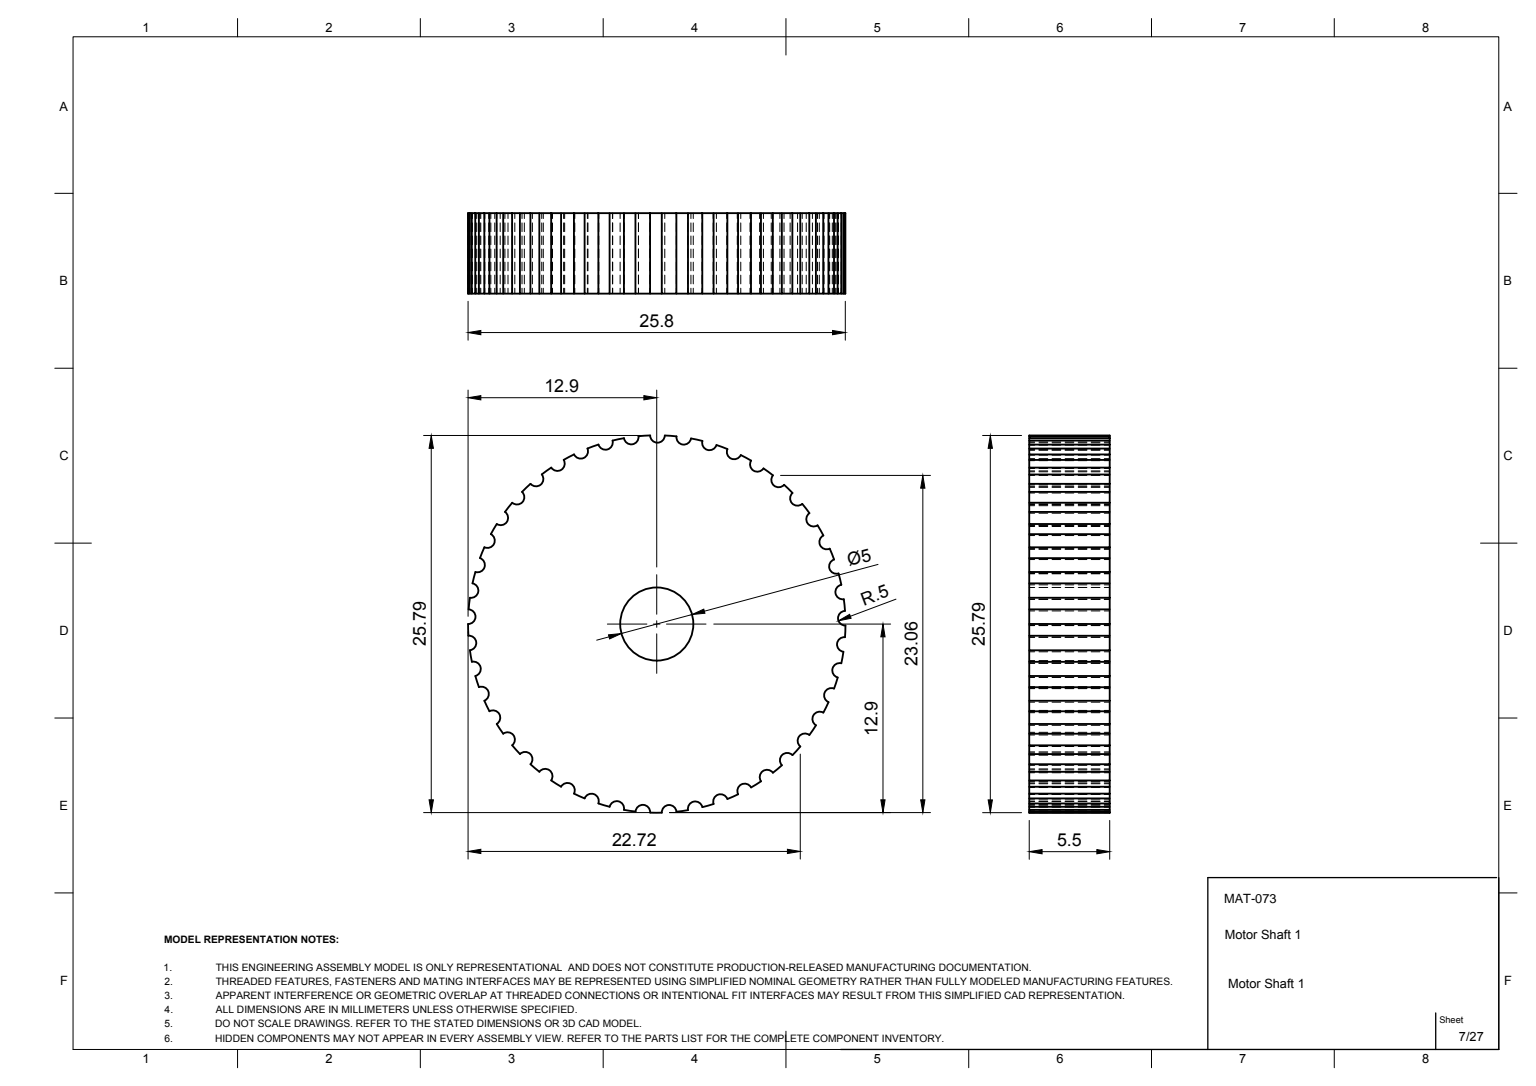
ISO-10303-21;
HEADER;
/* Generated by software containing ST-Developer
 * from STEP Tools, Inc. (www.steptools.com) 
 */

FILE_DESCRIPTION(
/* description */ ('CAx-IF Rec.Pracs.---Representation and Presentation of Product Manufa
cturing Information (PMI)---4.0---2014-10-13'),
/* implementation_level */ '2;1');

FILE_NAME(
/* name */ 'Motor Shaft 1.step',
/* time_stamp */ '2026-10-24T18:52:33-07:00',
/* author */ (''),
/* organization */ (''),
/* preprocessor_version */ 'ST-DEVELOPER v20.2',
/* originating_system */ 'Autodesk Translation Framework v15.17.0.0',
/* authorisation */ '');

FILE_SCHEMA (('AP242_MANAGED_MODEL_BASED_3D_ENGINEERING_MIM_LF { 1 0 10303 442 2 1 4 }'));
ENDSEC;

DATA;
#10=MECHANICAL_DESIGN_GEOMETRIC_PRESENTATION_REPRESENTATION('',(#418),#34876);
#352=SHAPE_REPRESENTATION_RELATIONSHIP('SRR','None',#34989,#385);
#385=ADVANCED_BREP_SHAPE_REPRESENTATION('',(#451),#34847);
#418=STYLED_ITEM('',(#35163),#451);
#451=MANIFOLD_SOLID_BREP('Motor Shaft 1',#19558);
#501=FACE_BOUND('',#6091,.T.);
#502=FACE_BOUND('',#6138,.T.);
#717=PLANE('',#20448);
#718=PLANE('',#20586);
#1387=LINE('',#29757,#2986);
#1388=LINE('',#29761,#2987);
#1389=LINE('',#29766,#2988);
#1390=LINE('',#29770,#2989);
#1391=LINE('',#29775,#2990);
#1392=LINE('',#29779,#2991);
#1393=LINE('',#29784,#2992);
#1394=LINE('',#29788,#2993);
#1395=LINE('',#29793,#2994);
#1396=LINE('',#29797,#2995);
#1397=LINE('',#29802,#2996);
#1398=LINE('',#29806,#2997);
#1399=LINE('',#29811,#2998);
#1400=LINE('',#29815,#2999);
#1401=LINE('',#29820,#3000);
#1402=LINE('',#29824,#3001);
#1403=LINE('',#29829,#3002);
#1404=LINE('',#29833,#3003);
#1405=LINE('',#29838,#3004);
#1406=LINE('',#29842,#3005);
#1407=LINE('',#29847,#3006);
#1408=LINE('',#29851,#3007);
#1409=LINE('',#29856,#3008);
#1410=LINE('',#29860,#3009);
#1411=LINE('',#29865,#3010);
#1412=LINE('',#29869,#3011);
#1413=LINE('',#29874,#3012);
#1414=LINE('',#29878,#3013);
#1415=LINE('',#29883,#3014);
#1416=LINE('',#29887,#3015);
#1417=LINE('',#29892,#3016);
#1418=LINE('',#29896,#3017);
#1419=LINE('',#29901,#3018);
#1420=LINE('',#29905,#3019);
#1421=LINE('',#29910,#3020);
#1422=LINE('',#29914,#3021);
#1423=LINE('',#29919,#3022);
#1424=LINE('',#29923,#3023);
#1425=LINE('',#29928,#3024);
#1426=LINE('',#29932,#3025);
#1427=LINE('',#29937,#3026);
#1428=LINE('',#29941,#3027);
#1429=LINE('',#29946,#3028);
#1430=LINE('',#29950,#3029);
#1431=LINE('',#29955,#3030);
#1432=LINE('',#29959,#3031);
#1433=LINE('',#29964,#3032);
#1434=LINE('',#29968,#3033);
#1435=LINE('',#29973,#3034);
#1436=LINE('',#29977,#3035);
#1437=LINE('',#29982,#3036);
#1438=LINE('',#29986,#3037);
#1439=LINE('',#29991,#3038);
#1440=LINE('',#29995,#3039);
#1441=LINE('',#30000,#3040);
#1442=LINE('',#30004,#3041);
#1443=LINE('',#30009,#3042);
#1444=LINE('',#30013,#3043);
#1445=LINE('',#30018,#3044);
#1446=LINE('',#30022,#3045);
#1447=LINE('',#30027,#3046);
#1448=LINE('',#30031,#3047);
#1449=LINE('',#30036,#3048);
#1450=LINE('',#30040,#3049);
#1451=LINE('',#30045,#3050);
#1452=LINE('',#30049,#3051);
#1453=LINE('',#30054,#3052);
#1454=LINE('',#30058,#3053);
#1455=LINE('',#30063,#3054);
#1456=LINE('',#30067,#3055);
#1457=LINE('',#30072,#3056);
#1458=LINE('',#30076,#3057);
#1459=LINE('',#30081,#3058);
#1460=LINE('',#30085,#3059);
#1461=LINE('',#30090,#3060);
#1462=LINE('',#30094,#3061);
#1463=LINE('',#30099,#3062);
#1464=LINE('',#30103,#3063);
#1465=LINE('',#30108,#3064);
#1466=LINE('',#30112,#3065);
#1467=LINE('',#30117,#3066);
#1468=LINE('',#30121,#3067);
#1469=LINE('',#30126,#3068);
#1470=LINE('',#30130,#3069);
#1471=LINE('',#30135,#3070);
#1472=LINE('',#30139,#3071);
#1473=LINE('',#30144,#3072);
#1474=LINE('',#30148,#3073);
#1475=LINE('',#30204,#3074);
#1476=LINE('',#30207,#3075);
#1477=LINE('',#30301,#3076);
#2986=VECTOR('',#23294,1.);
#2987=VECTOR('',#23297,1.);
#2988=VECTOR('',#23302,1.);
#2989=VECTOR('',#23305,1.);
#2990=VECTOR('',#23310,1.);
#2991=VECTOR('',#23313,1.);
#2992=VECTOR('',#23318,1.);
#2993=VECTOR('',#23321,1.);
#2994=VECTOR('',#23326,1.);
#2995=VECTOR('',#23329,1.);
#2996=VECTOR('',#23334,1.);
#2997=VECTOR('',#23337,1.);
#2998=VECTOR('',#23342,1.);
#2999=VECTOR('',#23345,1.);
#3000=VECTOR('',#23350,1.);
#3001=VECTOR('',#23353,1.);
#3002=VECTOR('',#23358,1.);
#3003=VECTOR('',#23361,1.);
#3004=VECTOR('',#23366,1.);
#3005=VECTOR('',#23369,1.);
#3006=VECTOR('',#23374,1.);
#3007=VECTOR('',#23377,1.);
#3008=VECTOR('',#23382,1.);
#3009=VECTOR('',#23385,1.);
#3010=VECTOR('',#23390,1.);
#3011=VECTOR('',#23393,1.);
#3012=VECTOR('',#23398,1.);
#3013=VECTOR('',#23401,1.);
#3014=VECTOR('',#23406,1.);
#3015=VECTOR('',#23409,1.);
#3016=VECTOR('',#23414,1.);
#3017=VECTOR('',#23417,1.);
#3018=VECTOR('',#23422,1.);
#3019=VECTOR('',#23425,1.);
#3020=VECTOR('',#23430,1.);
#3021=VECTOR('',#23433,1.);
#3022=VECTOR('',#23438,1.);
#3023=VECTOR('',#23441,1.);
#3024=VECTOR('',#23446,1.);
#3025=VECTOR('',#23449,1.);
#3026=VECTOR('',#23454,1.);
#3027=VECTOR('',#23457,1.);
#3028=VECTOR('',#23462,1.);
#3029=VECTOR('',#23465,1.);
#3030=VECTOR('',#23470,1.);
#3031=VECTOR('',#23473,1.);
#3032=VECTOR('',#23478,1.);
#3033=VECTOR('',#23481,1.);
#3034=VECTOR('',#23486,1.);
#3035=VECTOR('',#23489,1.);
#3036=VECTOR('',#23494,1.);
#3037=VECTOR('',#23497,1.);
#3038=VECTOR('',#23502,1.);
#3039=VECTOR('',#23505,1.);
#3040=VECTOR('',#23510,1.);
#3041=VECTOR('',#23513,1.);
#3042=VECTOR('',#23518,1.);
#3043=VECTOR('',#23521,1.);
#3044=VECTOR('',#23526,1.);
#3045=VECTOR('',#23529,1.);
#3046=VECTOR('',#23534,1.);
#3047=VECTOR('',#23537,1.);
#3048=VECTOR('',#23542,1.);
#3049=VECTOR('',#23545,1.);
#3050=VECTOR('',#23550,1.);
#3051=VECTOR('',#23553,1.);
#3052=VECTOR('',#23558,1.);
#3053=VECTOR('',#23561,1.);
#3054=VECTOR('',#23566,1.);
#3055=VECTOR('',#23569,1.);
#3056=VECTOR('',#23574,1.);
#3057=VECTOR('',#23577,1.);
#3058=VECTOR('',#23582,1.);
#3059=VECTOR('',#23585,1.);
#3060=VECTOR('',#23590,1.);
#3061=VECTOR('',#23593,1.);
#3062=VECTOR('',#23598,1.);
#3063=VECTOR('',#23601,1.);
#3064=VECTOR('',#23606,1.);
#3065=VECTOR('',#23609,1.);
#3066=VECTOR('',#23614,1.);
#3067=VECTOR('',#23617,1.);
#3068=VECTOR('',#23622,1.);
#3069=VECTOR('',#23625,1.);
#3070=VECTOR('',#23630,1.);
#3071=VECTOR('',#23633,1.);
#3072=VECTOR('',#23638,1.);
#3073=VECTOR('',#23641,1.);
#3074=VECTOR('',#23744,1.);
#3075=VECTOR('',#23747,1.);
#3076=VECTOR('',#23932,0.0025);
#4339=CYLINDRICAL_SURFACE('',#20316,0.0005);
#4340=CYLINDRICAL_SURFACE('',#20319,0.0005);
#4341=CYLINDRICAL_SURFACE('',#20322,0.0005);
#4342=CYLINDRICAL_SURFACE('',#20325,0.0005);
#4343=CYLINDRICAL_SURFACE('',#20328,0.0005);
#4344=CYLINDRICAL_SURFACE('',#20331,0.0005);
#4345=CYLINDRICAL_SURFACE('',#20334,0.0005);
#4346=CYLINDRICAL_SURFACE('',#20337,0.0005);
#4347=CYLINDRICAL_SURFACE('',#20340,0.0005);
#4348=CYLINDRICAL_SURFACE('',#20343,0.0005);
#4349=CYLINDRICAL_SURFACE('',#20346,0.0005);
#4350=CYLINDRICAL_SURFACE('',#20349,0.0005);
#4351=CYLINDRICAL_SURFACE('',#20352,0.0005);
#4352=CYLINDRICAL_SURFACE('',#20355,0.0005);
#4353=CYLINDRICAL_SURFACE('',#20358,0.0005);
#4354=CYLINDRICAL_SURFACE('',#20361,0.0005);
#4355=CYLINDRICAL_SURFACE('',#20364,0.0005);
#4356=CYLINDRICAL_SURFACE('',#20367,0.0005);
#4357=CYLINDRICAL_SURFACE('',#20370,0.0005);
#4358=CYLINDRICAL_SURFACE('',#20373,0.0005);
#4359=CYLINDRICAL_SURFACE('',#20376,0.0005);
#4360=CYLINDRICAL_SURFACE('',#20379,0.0005);
#4361=CYLINDRICAL_SURFACE('',#20382,0.0005);
#4362=CYLINDRICAL_SURFACE('',#20385,0.0005);
#4363=CYLINDRICAL_SURFACE('',#20388,0.0005);
#4364=CYLINDRICAL_SURFACE('',#20391,0.0005);
#4365=CYLINDRICAL_SURFACE('',#20394,0.0005);
#4366=CYLINDRICAL_SURFACE('',#20397,0.0005);
#4367=CYLINDRICAL_SURFACE('',#20400,0.0005);
#4368=CYLINDRICAL_SURFACE('',#20403,0.0005);
#4369=CYLINDRICAL_SURFACE('',#20406,0.0005);
#4370=CYLINDRICAL_SURFACE('',#20409,0.0005);
#4371=CYLINDRICAL_SURFACE('',#20412,0.0005);
#4372=CYLINDRICAL_SURFACE('',#20415,0.0005);
#4373=CYLINDRICAL_SURFACE('',#20418,0.0005);
#4374=CYLINDRICAL_SURFACE('',#20421,0.0005);
#4375=CYLINDRICAL_SURFACE('',#20424,0.0005);
#4376=CYLINDRICAL_SURFACE('',#20427,0.0005);
#4377=CYLINDRICAL_SURFACE('',#20430,0.0005);
#4378=CYLINDRICAL_SURFACE('',#20433,0.0005);
#4379=CYLINDRICAL_SURFACE('',#20436,0.0005);
#4380=CYLINDRICAL_SURFACE('',#20439,0.0005);
#4381=CYLINDRICAL_SURFACE('',#20442,0.0005);
#4382=CYLINDRICAL_SURFACE('',#20445,0.0005);
#4383=CYLINDRICAL_SURFACE('',#20496,0.0129);
#4384=CYLINDRICAL_SURFACE('',#20498,0.0129);
#4385=CYLINDRICAL_SURFACE('',#20500,0.0129);
#4386=CYLINDRICAL_SURFACE('',#20502,0.0129);
#4387=CYLINDRICAL_SURFACE('',#20504,0.0129);
#4388=CYLINDRICAL_SURFACE('',#20506,0.0129);
#4389=CYLINDRICAL_SURFACE('',#20508,0.0129);
#4390=CYLINDRICAL_SURFACE('',#20510,0.0129);
#4391=CYLINDRICAL_SURFACE('',#20512,0.0129);
#4392=CYLINDRICAL_SURFACE('',#20514,0.0129);
#4393=CYLINDRICAL_SURFACE('',#20516,0.0129);
#4394=CYLINDRICAL_SURFACE('',#20518,0.0129);
#4395=CYLINDRICAL_SURFACE('',#20520,0.0129);
#4396=CYLINDRICAL_SURFACE('',#20522,0.0129);
#4397=CYLINDRICAL_SURFACE('',#20524,0.0129);
#4398=CYLINDRICAL_SURFACE('',#20526,0.0129);
#4399=CYLINDRICAL_SURFACE('',#20528,0.0129);
#4400=CYLINDRICAL_SURFACE('',#20530,0.0129);
#4401=CYLINDRICAL_SURFACE('',#20532,0.0129);
#4402=CYLINDRICAL_SURFACE('',#20534,0.0129);
#4403=CYLINDRICAL_SURFACE('',#20536,0.0129);
#4404=CYLINDRICAL_SURFACE('',#20538,0.0129);
#4405=CYLINDRICAL_SURFACE('',#20540,0.0129);
#4406=CYLINDRICAL_SURFACE('',#20542,0.0129);
#4407=CYLINDRICAL_SURFACE('',#20544,0.0129);
#4408=CYLINDRICAL_SURFACE('',#20546,0.0129);
#4409=CYLINDRICAL_SURFACE('',#20548,0.0129);
#4410=CYLINDRICAL_SURFACE('',#20550,0.0129);
#4411=CYLINDRICAL_SURFACE('',#20552,0.0129);
#4412=CYLINDRICAL_SURFACE('',#20554,0.0129);
#4413=CYLINDRICAL_SURFACE('',#20556,0.0129);
#4414=CYLINDRICAL_SURFACE('',#20558,0.0129);
#4415=CYLINDRICAL_SURFACE('',#20560,0.0129);
#4416=CYLINDRICAL_SURFACE('',#20562,0.0129);
#4417=CYLINDRICAL_SURFACE('',#20564,0.0129);
#4418=CYLINDRICAL_SURFACE('',#20566,0.0129);
#4419=CYLINDRICAL_SURFACE('',#20568,0.0129);
#4420=CYLINDRICAL_SURFACE('',#20570,0.0129);
#4421=CYLINDRICAL_SURFACE('',#20572,0.0129);
#4422=CYLINDRICAL_SURFACE('',#20574,0.0129);
#4423=CYLINDRICAL_SURFACE('',#20576,0.0129);
#4424=CYLINDRICAL_SURFACE('',#20578,0.0129);
#4425=CYLINDRICAL_SURFACE('',#20580,0.0129);
#4426=CYLINDRICAL_SURFACE('',#20582,0.0129);
#4427=CYLINDRICAL_SURFACE('',#20584,0.0005);
#4428=CYLINDRICAL_SURFACE('',#20589,0.0129);
#4429=CYLINDRICAL_SURFACE('',#20590,0.0025);
#4980=FACE_OUTER_BOUND('',#6046,.T.);
#4981=FACE_OUTER_BOUND('',#6047,.T.);
#4982=FACE_OUTER_BOUND('',#6048,.T.);
#4983=FACE_OUTER_BOUND('',#6049,.T.);
#4984=FACE_OUTER_BOUND('',#6050,.T.);
#4985=FACE_OUTER_BOUND('',#6051,.T.);
#4986=FACE_OUTER_BOUND('',#6052,.T.);
#4987=FACE_OUTER_BOUND('',#6053,.T.);
#4988=FACE_OUTER_BOUND('',#6054,.T.);
#4989=FACE_OUTER_BOUND('',#6055,.T.);
#4990=FACE_OUTER_BOUND('',#6056,.T.);
#4991=FACE_OUTER_BOUND('',#6057,.T.);
#4992=FACE_OUTER_BOUND('',#6058,.T.);
#4993=FACE_OUTER_BOUND('',#6059,.T.);
#4994=FACE_OUTER_BOUND('',#6060,.T.);
#4995=FACE_OUTER_BOUND('',#6061,.T.);
#4996=FACE_OUTER_BOUND('',#6062,.T.);
#4997=FACE_OUTER_BOUND('',#6063,.T.);
#4998=FACE_OUTER_BOUND('',#6064,.T.);
#4999=FACE_OUTER_BOUND('',#6065,.T.);
#5000=FACE_OUTER_BOUND('',#6066,.T.);
#5001=FACE_OUTER_BOUND('',#6067,.T.);
#5002=FACE_OUTER_BOUND('',#6068,.T.);
#5003=FACE_OUTER_BOUND('',#6069,.T.);
#5004=FACE_OUTER_BOUND('',#6070,.T.);
#5005=FACE_OUTER_BOUND('',#6071,.T.);
#5006=FACE_OUTER_BOUND('',#6072,.T.);
#5007=FACE_OUTER_BOUND('',#6073,.T.);
#5008=FACE_OUTER_BOUND('',#6074,.T.);
#5009=FACE_OUTER_BOUND('',#6075,.T.);
#5010=FACE_OUTER_BOUND('',#6076,.T.);
#5011=FACE_OUTER_BOUND('',#6077,.T.);
#5012=FACE_OUTER_BOUND('',#6078,.T.);
#5013=FACE_OUTER_BOUND('',#6079,.T.);
#5014=FACE_OUTER_BOUND('',#6080,.T.);
#5015=FACE_OUTER_BOUND('',#6081,.T.);
#5016=FACE_OUTER_BOUND('',#6082,.T.);
#5017=FACE_OUTER_BOUND('',#6083,.T.);
#5018=FACE_OUTER_BOUND('',#6084,.T.);
#5019=FACE_OUTER_BOUND('',#6085,.T.);
#5020=FACE_OUTER_BOUND('',#6086,.T.);
#5021=FACE_OUTER_BOUND('',#6087,.T.);
#5022=FACE_OUTER_BOUND('',#6088,.T.);
#5023=FACE_OUTER_BOUND('',#6089,.T.);
#5024=FACE_OUTER_BOUND('',#6090,.T.);
#5025=FACE_OUTER_BOUND('',#6092,.T.);
#5026=FACE_OUTER_BOUND('',#6093,.T.);
#5027=FACE_OUTER_BOUND('',#6094,.T.);
#5028=FACE_OUTER_BOUND('',#6095,.T.);
#5029=FACE_OUTER_BOUND('',#6096,.T.);
#5030=FACE_OUTER_BOUND('',#6097,.T.);
#5031=FACE_OUTER_BOUND('',#6098,.T.);
#5032=FACE_OUTER_BOUND('',#6099,.T.);
#5033=FACE_OUTER_BOUND('',#6100,.T.);
#5034=FACE_OUTER_BOUND('',#6101,.T.);
#5035=FACE_OUTER_BOUND('',#6102,.T.);
#5036=FACE_OUTER_BOUND('',#6103,.T.);
#5037=FACE_OUTER_BOUND('',#6104,.T.);
#5038=FACE_OUTER_BOUND('',#6105,.T.);
#5039=FACE_OUTER_BOUND('',#6106,.T.);
#5040=FACE_OUTER_BOUND('',#6107,.T.);
#5041=FACE_OUTER_BOUND('',#6108,.T.);
#5042=FACE_OUTER_BOUND('',#6109,.T.);
#5043=FACE_OUTER_BOUND('',#6110,.T.);
#5044=FACE_OUTER_BOUND('',#6111,.T.);
#5045=FACE_OUTER_BOUND('',#6112,.T.);
#5046=FACE_OUTER_BOUND('',#6113,.T.);
#5047=FACE_OUTER_BOUND('',#6114,.T.);
#5048=FACE_OUTER_BOUND('',#6115,.T.);
#5049=FACE_OUTER_BOUND('',#6116,.T.);
#5050=FACE_OUTER_BOUND('',#6117,.T.);
#5051=FACE_OUTER_BOUND('',#6118,.T.);
#5052=FACE_OUTER_BOUND('',#6119,.T.);
#5053=FACE_OUTER_BOUND('',#6120,.T.);
#5054=FACE_OUTER_BOUND('',#6121,.T.);
#5055=FACE_OUTER_BOUND('',#6122,.T.);
#5056=FACE_OUTER_BOUND('',#6123,.T.);
#5057=FACE_OUTER_BOUND('',#6124,.T.);
#5058=FACE_OUTER_BOUND('',#6125,.T.);
#5059=FACE_OUTER_BOUND('',#6126,.T.);
#5060=FACE_OUTER_BOUND('',#6127,.T.);
#5061=FACE_OUTER_BOUND('',#6128,.T.);
#5062=FACE_OUTER_BOUND('',#6129,.T.);
#5063=FACE_OUTER_BOUND('',#6130,.T.);
#5064=FACE_OUTER_BOUND('',#6131,.T.);
#5065=FACE_OUTER_BOUND('',#6132,.T.);
#5066=FACE_OUTER_BOUND('',#6133,.T.);
#5067=FACE_OUTER_BOUND('',#6134,.T.);
#5068=FACE_OUTER_BOUND('',#6135,.T.);
#5069=FACE_OUTER_BOUND('',#6136,.T.);
#5070=FACE_OUTER_BOUND('',#6137,.T.);
#5071=FACE_OUTER_BOUND('',#6139,.T.);
#5072=FACE_OUTER_BOUND('',#6140,.T.);
#6046=EDGE_LOOP('',(#13790,#13791,#13792,#13793));
#6047=EDGE_LOOP('',(#13794,#13795,#13796,#13797));
#6048=EDGE_LOOP('',(#13798,#13799,#13800,#13801));
#6049=EDGE_LOOP('',(#13802,#13803,#13804,#13805));
#6050=EDGE_LOOP('',(#13806,#13807,#13808,#13809));
#6051=EDGE_LOOP('',(#13810,#13811,#13812,#13813));
#6052=EDGE_LOOP('',(#13814,#13815,#13816,#13817));
#6053=EDGE_LOOP('',(#13818,#13819,#13820,#13821));
#6054=EDGE_LOOP('',(#13822,#13823,#13824,#13825));
#6055=EDGE_LOOP('',(#13826,#13827,#13828,#13829));
#6056=EDGE_LOOP('',(#13830,#13831,#13832,#13833));
#6057=EDGE_LOOP('',(#13834,#13835,#13836,#13837));
#6058=EDGE_LOOP('',(#13838,#13839,#13840,#13841));
#6059=EDGE_LOOP('',(#13842,#13843,#13844,#13845));
#6060=EDGE_LOOP('',(#13846,#13847,#13848,#13849));
#6061=EDGE_LOOP('',(#13850,#13851,#13852,#13853));
#6062=EDGE_LOOP('',(#13854,#13855,#13856,#13857));
#6063=EDGE_LOOP('',(#13858,#13859,#13860,#13861));
#6064=EDGE_LOOP('',(#13862,#13863,#13864,#13865));
#6065=EDGE_LOOP('',(#13866,#13867,#13868,#13869));
#6066=EDGE_LOOP('',(#13870,#13871,#13872,#13873));
#6067=EDGE_LOOP('',(#13874,#13875,#13876,#13877));
#6068=EDGE_LOOP('',(#13878,#13879,#13880,#13881));
#6069=EDGE_LOOP('',(#13882,#13883,#13884,#13885));
#6070=EDGE_LOOP('',(#13886,#13887,#13888,#13889));
#6071=EDGE_LOOP('',(#13890,#13891,#13892,#13893));
#6072=EDGE_LOOP('',(#13894,#13895,#13896,#13897));
#6073=EDGE_LOOP('',(#13898,#13899,#13900,#13901));
#6074=EDGE_LOOP('',(#13902,#13903,#13904,#13905));
#6075=EDGE_LOOP('',(#13906,#13907,#13908,#13909));
#6076=EDGE_LOOP('',(#13910,#13911,#13912,#13913));
#6077=EDGE_LOOP('',(#13914,#13915,#13916,#13917));
#6078=EDGE_LOOP('',(#13918,#13919,#13920,#13921));
#6079=EDGE_LOOP('',(#13922,#13923,#13924,#13925));
#6080=EDGE_LOOP('',(#13926,#13927,#13928,#13929));
#6081=EDGE_LOOP('',(#13930,#13931,#13932,#13933));
#6082=EDGE_LOOP('',(#13934,#13935,#13936,#13937));
#6083=EDGE_LOOP('',(#13938,#13939,#13940,#13941));
#6084=EDGE_LOOP('',(#13942,#13943,#13944,#13945));
#6085=EDGE_LOOP('',(#13946,#13947,#13948,#13949));
#6086=EDGE_LOOP('',(#13950,#13951,#13952,#13953));
#6087=EDGE_LOOP('',(#13954,#13955,#13956,#13957));
#6088=EDGE_LOOP('',(#13958,#13959,#13960,#13961));
#6089=EDGE_LOOP('',(#13962,#13963,#13964,#13965));
#6090=EDGE_LOOP('',(#13966,#13967,#13968,#13969,#13970,#13971,#13972,#13973,
#13974,#13975,#13976,#13977,#13978,#13979,#13980,#13981,#13982,#13983,#13984,
#13985,#13986,#13987,#13988,#13989,#13990,#13991,#13992,#13993,#13994,#13995,
#13996,#13997,#13998,#13999,#14000,#14001,#14002,#14003,#14004,#14005,#14006,
#14007,#14008,#14009,#14010,#14011,#14012,#14013,#14014,#14015,#14016,#14017,
#14018,#14019,#14020,#14021,#14022,#14023,#14024,#14025,#14026,#14027,#14028,
#14029,#14030,#14031,#14032,#14033,#14034,#14035,#14036,#14037,#14038,#14039,
#14040,#14041,#14042,#14043,#14044,#14045,#14046,#14047,#14048,#14049,#14050,
#14051,#14052,#14053,#14054,#14055));
#6091=EDGE_LOOP('',(#14056));
#6092=EDGE_LOOP('',(#14057,#14058,#14059,#14060));
#6093=EDGE_LOOP('',(#14061,#14062,#14063,#14064));
#6094=EDGE_LOOP('',(#14065,#14066,#14067,#14068));
#6095=EDGE_LOOP('',(#14069,#14070,#14071,#14072));
#6096=EDGE_LOOP('',(#14073,#14074,#14075,#14076));
#6097=EDGE_LOOP('',(#14077,#14078,#14079,#14080));
#6098=EDGE_LOOP('',(#14081,#14082,#14083,#14084));
#6099=EDGE_LOOP('',(#14085,#14086,#14087,#14088));
#6100=EDGE_LOOP('',(#14089,#14090,#14091,#14092));
#6101=EDGE_LOOP('',(#14093,#14094,#14095,#14096));
#6102=EDGE_LOOP('',(#14097,#14098,#14099,#14100));
#6103=EDGE_LOOP('',(#14101,#14102,#14103,#14104));
#6104=EDGE_LOOP('',(#14105,#14106,#14107,#14108));
#6105=EDGE_LOOP('',(#14109,#14110,#14111,#14112));
#6106=EDGE_LOOP('',(#14113,#14114,#14115,#14116));
#6107=EDGE_LOOP('',(#14117,#14118,#14119,#14120));
#6108=EDGE_LOOP('',(#14121,#14122,#14123,#14124));
#6109=EDGE_LOOP('',(#14125,#14126,#14127,#14128));
#6110=EDGE_LOOP('',(#14129,#14130,#14131,#14132));
#6111=EDGE_LOOP('',(#14133,#14134,#14135,#14136));
#6112=EDGE_LOOP('',(#14137,#14138,#14139,#14140));
#6113=EDGE_LOOP('',(#14141,#14142,#14143,#14144));
#6114=EDGE_LOOP('',(#14145,#14146,#14147,#14148));
#6115=EDGE_LOOP('',(#14149,#14150,#14151,#14152));
#6116=EDGE_LOOP('',(#14153,#14154,#14155,#14156));
#6117=EDGE_LOOP('',(#14157,#14158,#14159,#14160));
#6118=EDGE_LOOP('',(#14161,#14162,#14163,#14164));
#6119=EDGE_LOOP('',(#14165,#14166,#14167,#14168));
#6120=EDGE_LOOP('',(#14169,#14170,#14171,#14172));
#6121=EDGE_LOOP('',(#14173,#14174,#14175,#14176));
#6122=EDGE_LOOP('',(#14177,#14178,#14179,#14180));
#6123=EDGE_LOOP('',(#14181,#14182,#14183,#14184));
#6124=EDGE_LOOP('',(#14185,#14186,#14187,#14188));
#6125=EDGE_LOOP('',(#14189,#14190,#14191,#14192));
#6126=EDGE_LOOP('',(#14193,#14194,#14195,#14196));
#6127=EDGE_LOOP('',(#14197,#14198,#14199,#14200));
#6128=EDGE_LOOP('',(#14201,#14202,#14203,#14204));
#6129=EDGE_LOOP('',(#14205,#14206,#14207,#14208));
#6130=EDGE_LOOP('',(#14209,#14210,#14211,#14212));
#6131=EDGE_LOOP('',(#14213,#14214,#14215,#14216));
#6132=EDGE_LOOP('',(#14217,#14218,#14219,#14220));
#6133=EDGE_LOOP('',(#14221,#14222,#14223,#14224));
#6134=EDGE_LOOP('',(#14225,#14226,#14227,#14228));
#6135=EDGE_LOOP('',(#14229,#14230,#14231,#14232));
#6136=EDGE_LOOP('',(#14233,#14234,#14235,#14236));
#6137=EDGE_LOOP('',(#14237,#14238,#14239,#14240,#14241,#14242,#14243,#14244,
#14245,#14246,#14247,#14248,#14249,#14250,#14251,#14252,#14253,#14254,#14255,
#14256,#14257,#14258,#14259,#14260,#14261,#14262,#14263,#14264,#14265,#14266,
#14267,#14268,#14269,#14270,#14271,#14272,#14273,#14274,#14275,#14276,#14277,
#14278,#14279,#14280,#14281,#14282,#14283,#14284,#14285,#14286,#14287,#14288,
#14289,#14290,#14291,#14292,#14293,#14294,#14295,#14296,#14297,#14298,#14299,
#14300,#14301,#14302,#14303,#14304,#14305,#14306,#14307,#14308,#14309,#14310,
#14311,#14312,#14313,#14314,#14315,#14316,#14317,#14318,#14319,#14320,#14321,
#14322,#14323,#14324,#14325,#14326));
#6138=EDGE_LOOP('',(#14327));
#6139=EDGE_LOOP('',(#14328,#14329,#14330,#14331));
#6140=EDGE_LOOP('',(#14332,#14333,#14334,#14335));
#7101=CIRCLE('',#20317,0.000500000000011295);
#7102=CIRCLE('',#20318,0.000500000000011295);
#7103=CIRCLE('',#20320,0.000500000000012369);
#7104=CIRCLE('',#20321,0.000500000000012369);
#7105=CIRCLE('',#20323,0.000500000000013203);
#7106=CIRCLE('',#20324,0.000500000000013203);
#7107=CIRCLE('',#20326,0.00050000000001378);
#7108=CIRCLE('',#20327,0.00050000000001378);
#7109=CIRCLE('',#20329,0.000500000000014088);
#7110=CIRCLE('',#20330,0.000500000000014088);
#7111=CIRCLE('',#20332,0.000500000000014123);
#7112=CIRCLE('',#20333,0.000500000000014123);
#7113=CIRCLE('',#20335,0.000500000000013882);
#7114=CIRCLE('',#20336,0.000500000000013882);
#7115=CIRCLE('',#20338,0.000500000000013372);
#7116=CIRCLE('',#20339,0.000500000000013372);
#7117=CIRCLE('',#20341,0.000500000000012601);
#7118=CIRCLE('',#20342,0.000500000000012601);
#7119=CIRCLE('',#20344,0.000500000000011585);
#7120=CIRCLE('',#20345,0.000500000000011585);
#7121=CIRCLE('',#20347,0.000500000000010343);
#7122=CIRCLE('',#20348,0.000500000000010343);
#7123=CIRCLE('',#20350,0.000500000000010991);
#7124=CIRCLE('',#20351,0.000500000000010991);
#7125=CIRCLE('',#20353,0.000500000000012122);
#7126=CIRCLE('',#20354,0.000500000000012122);
#7127=CIRCLE('',#20356,0.000500000000013018);
#7128=CIRCLE('',#20357,0.000500000000013018);
#7129=CIRCLE('',#20359,0.00050000000001366);
#7130=CIRCLE('',#20360,0.00050000000001366);
#7131=CIRCLE('',#20362,0.000500000000014037);
#7132=CIRCLE('',#20363,0.000500000000014037);
#7133=CIRCLE('',#20365,0.00050000000001414);
#7134=CIRCLE('',#20366,0.00050000000001414);
#7135=CIRCLE('',#20368,0.000500000000013968);
#7136=CIRCLE('',#20369,0.000500000000013968);
#7137=CIRCLE('',#20371,0.000500000000013524);
#7138=CIRCLE('',#20372,0.000500000000013524);
#7139=CIRCLE('',#20374,0.000500000000012817);
#7140=CIRCLE('',#20375,0.000500000000012817);
#7141=CIRCLE('',#20377,0.000500000000011861);
#7142=CIRCLE('',#20378,0.000500000000011861);
#7143=CIRCLE('',#20380,0.000500000000010673);
#7144=CIRCLE('',#20381,0.000500000000010673);
#7145=CIRCLE('',#20383,0.000500000000010673);
#7146=CIRCLE('',#20384,0.000500000000010673);
#7147=CIRCLE('',#20386,0.000500000000011861);
#7148=CIRCLE('',#20387,0.000500000000011861);
#7149=CIRCLE('',#20389,0.000500000000012817);
#7150=CIRCLE('',#20390,0.000500000000012817);
#7151=CIRCLE('',#20392,0.000500000000013524);
#7152=CIRCLE('',#20393,0.000500000000013524);
#7153=CIRCLE('',#20395,0.000500000000013968);
#7154=CIRCLE('',#20396,0.000500000000013968);
#7155=CIRCLE('',#20398,0.00050000000001414);
#7156=CIRCLE('',#20399,0.00050000000001414);
#7157=CIRCLE('',#20401,0.000500000000014037);
#7158=CIRCLE('',#20402,0.000500000000014037);
#7159=CIRCLE('',#20404,0.00050000000001366);
#7160=CIRCLE('',#20405,0.00050000000001366);
#7161=CIRCLE('',#20407,0.000500000000013018);
#7162=CIRCLE('',#20408,0.000500000000013018);
#7163=CIRCLE('',#20410,0.000500000000012122);
#7164=CIRCLE('',#20411,0.000500000000012122);
#7165=CIRCLE('',#20413,0.000500000000010991);
#7166=CIRCLE('',#20414,0.000500000000010991);
#7167=CIRCLE('',#20416,0.000500000000010343);
#7168=CIRCLE('',#20417,0.000500000000010343);
#7169=CIRCLE('',#20419,0.000500000000011585);
#7170=CIRCLE('',#20420,0.000500000000011585);
#7171=CIRCLE('',#20422,0.000500000000012601);
#7172=CIRCLE('',#20423,0.000500000000012601);
#7173=CIRCLE('',#20425,0.000500000000013372);
#7174=CIRCLE('',#20426,0.000500000000013372);
#7175=CIRCLE('',#20428,0.000500000000013882);
#7176=CIRCLE('',#20429,0.000500000000013882);
#7177=CIRCLE('',#20431,0.000500000000014123);
#7178=CIRCLE('',#20432,0.000500000000014123);
#7179=CIRCLE('',#20434,0.000500000000014088);
#7180=CIRCLE('',#20435,0.000500000000014088);
#7181=CIRCLE('',#20437,0.00050000000001378);
#7182=CIRCLE('',#20438,0.00050000000001378);
#7183=CIRCLE('',#20440,0.000500000000013203);
#7184=CIRCLE('',#20441,0.000500000000013203);
#7185=CIRCLE('',#20443,0.000500000000012369);
#7186=CIRCLE('',#20444,0.000500000000012369);
#7187=CIRCLE('',#20446,0.000500000000011295);
#7188=CIRCLE('',#20447,0.000500000000011295);
#7189=CIRCLE('',#20449,0.01290000000001);
#7190=CIRCLE('',#20450,0.00050000000001);
#7191=CIRCLE('',#20451,0.01290000000001);
#7192=CIRCLE('',#20452,0.01290000000001);
#7193=CIRCLE('',#20453,0.01290000000001);
#7194=CIRCLE('',#20454,0.01290000000001);
#7195=CIRCLE('',#20455,0.01290000000001);
#7196=CIRCLE('',#20456,0.01290000000001);
#7197=CIRCLE('',#20457,0.01290000000001);
#7198=CIRCLE('',#20458,0.01290000000001);
#7199=CIRCLE('',#20459,0.01290000000001);
#7200=CIRCLE('',#20460,0.01290000000001);
#7201=CIRCLE('',#20461,0.01290000000001);
#7202=CIRCLE('',#20462,0.01290000000001);
#7203=CIRCLE('',#20463,0.01290000000001);
#7204=CIRCLE('',#20464,0.01290000000001);
#7205=CIRCLE('',#20465,0.01290000000001);
#7206=CIRCLE('',#20466,0.01290000000001);
#7207=CIRCLE('',#20467,0.01290000000001);
#7208=CIRCLE('',#20468,0.01290000000001);
#7209=CIRCLE('',#20469,0.01290000000001);
#7210=CIRCLE('',#20470,0.01290000000001);
#7211=CIRCLE('',#20471,0.01290000000001);
#7212=CIRCLE('',#20472,0.01290000000001);
#7213=CIRCLE('',#20473,0.01290000000001);
#7214=CIRCLE('',#20474,0.01290000000001);
#7215=CIRCLE('',#20475,0.01290000000001);
#7216=CIRCLE('',#20476,0.01290000000001);
#7217=CIRCLE('',#20477,0.01290000000001);
#7218=CIRCLE('',#20478,0.01290000000001);
#7219=CIRCLE('',#20479,0.01290000000001);
#7220=CIRCLE('',#20480,0.01290000000001);
#7221=CIRCLE('',#20481,0.01290000000001);
#7222=CIRCLE('',#20482,0.01290000000001);
#7223=CIRCLE('',#20483,0.01290000000001);
#7224=CIRCLE('',#20484,0.01290000000001);
#7225=CIRCLE('',#20485,0.01290000000001);
#7226=CIRCLE('',#20486,0.01290000000001);
#7227=CIRCLE('',#20487,0.01290000000001);
#7228=CIRCLE('',#20488,0.01290000000001);
#7229=CIRCLE('',#20489,0.01290000000001);
#7230=CIRCLE('',#20490,0.01290000000001);
#7231=CIRCLE('',#20491,0.01290000000001);
#7232=CIRCLE('',#20492,0.01290000000001);
#7233=CIRCLE('',#20493,0.01290000000001);
#7234=CIRCLE('',#20494,0.01290000000001);
#7235=CIRCLE('',#20495,0.00250000000001);
#7236=CIRCLE('',#20497,0.01290000000001);
#7237=CIRCLE('',#20499,0.01290000000001);
#7238=CIRCLE('',#20501,0.01290000000001);
#7239=CIRCLE('',#20503,0.01290000000001);
#7240=CIRCLE('',#20505,0.01290000000001);
#7241=CIRCLE('',#20507,0.01290000000001);
#7242=CIRCLE('',#20509,0.01290000000001);
#7243=CIRCLE('',#20511,0.01290000000001);
#7244=CIRCLE('',#20513,0.01290000000001);
#7245=CIRCLE('',#20515,0.01290000000001);
#7246=CIRCLE('',#20517,0.01290000000001);
#7247=CIRCLE('',#20519,0.01290000000001);
#7248=CIRCLE('',#20521,0.01290000000001);
#7249=CIRCLE('',#20523,0.01290000000001);
#7250=CIRCLE('',#20525,0.01290000000001);
#7251=CIRCLE('',#20527,0.01290000000001);
#7252=CIRCLE('',#20529,0.01290000000001);
#7253=CIRCLE('',#20531,0.01290000000001);
#7254=CIRCLE('',#20533,0.01290000000001);
#7255=CIRCLE('',#20535,0.01290000000001);
#7256=CIRCLE('',#20537,0.01290000000001);
#7257=CIRCLE('',#20539,0.01290000000001);
#7258=CIRCLE('',#20541,0.01290000000001);
#7259=CIRCLE('',#20543,0.01290000000001);
#7260=CIRCLE('',#20545,0.01290000000001);
#7261=CIRCLE('',#20547,0.01290000000001);
#7262=CIRCLE('',#20549,0.01290000000001);
#7263=CIRCLE('',#20551,0.01290000000001);
#7264=CIRCLE('',#20553,0.01290000000001);
#7265=CIRCLE('',#20555,0.01290000000001);
#7266=CIRCLE('',#20557,0.01290000000001);
#7267=CIRCLE('',#20559,0.01290000000001);
#7268=CIRCLE('',#20561,0.01290000000001);
#7269=CIRCLE('',#20563,0.01290000000001);
#7270=CIRCLE('',#20565,0.01290000000001);
#7271=CIRCLE('',#20567,0.01290000000001);
#7272=CIRCLE('',#20569,0.01290000000001);
#7273=CIRCLE('',#20571,0.01290000000001);
#7274=CIRCLE('',#20573,0.01290000000001);
#7275=CIRCLE('',#20575,0.01290000000001);
#7276=CIRCLE('',#20577,0.01290000000001);
#7277=CIRCLE('',#20579,0.01290000000001);
#7278=CIRCLE('',#20581,0.01290000000001);
#7279=CIRCLE('',#20583,0.01290000000001);
#7280=CIRCLE('',#20585,0.00050000000001);
#7281=CIRCLE('',#20587,0.01290000000001);
#7282=CIRCLE('',#20588,0.00250000000001);
#8399=VERTEX_POINT('',#29755);
#8400=VERTEX_POINT('',#29756);
#8401=VERTEX_POINT('',#29758);
#8402=VERTEX_POINT('',#29760);
#8403=VERTEX_POINT('',#29764);
#8404=VERTEX_POINT('',#29765);
#8405=VERTEX_POINT('',#29767);
#8406=VERTEX_POINT('',#29769);
#8407=VERTEX_POINT('',#29773);
#8408=VERTEX_POINT('',#29774);
#8409=VERTEX_POINT('',#29776);
#8410=VERTEX_POINT('',#29778);
#8411=VERTEX_POINT('',#29782);
#8412=VERTEX_POINT('',#29783);
#8413=VERTEX_POINT('',#29785);
#8414=VERTEX_POINT('',#29787);
#8415=VERTEX_POINT('',#29791);
#8416=VERTEX_POINT('',#29792);
#8417=VERTEX_POINT('',#29794);
#8418=VERTEX_POINT('',#29796);
#8419=VERTEX_POINT('',#29800);
#8420=VERTEX_POINT('',#29801);
#8421=VERTEX_POINT('',#29803);
#8422=VERTEX_POINT('',#29805);
#8423=VERTEX_POINT('',#29809);
#8424=VERTEX_POINT('',#29810);
#8425=VERTEX_POINT('',#29812);
#8426=VERTEX_POINT('',#29814);
#8427=VERTEX_POINT('',#29818);
#8428=VERTEX_POINT('',#29819);
#8429=VERTEX_POINT('',#29821);
#8430=VERTEX_POINT('',#29823);
#8431=VERTEX_POINT('',#29827);
#8432=VERTEX_POINT('',#29828);
#8433=VERTEX_POINT('',#29830);
#8434=VERTEX_POINT('',#29832);
#8435=VERTEX_POINT('',#29836);
#8436=VERTEX_POINT('',#29837);
#8437=VERTEX_POINT('',#29839);
#8438=VERTEX_POINT('',#29841);
#8439=VERTEX_POINT('',#29845);
#8440=VERTEX_POINT('',#29846);
#8441=VERTEX_POINT('',#29848);
#8442=VERTEX_POINT('',#29850);
#8443=VERTEX_POINT('',#29854);
#8444=VERTEX_POINT('',#29855);
#8445=VERTEX_POINT('',#29857);
#8446=VERTEX_POINT('',#29859);
#8447=VERTEX_POINT('',#29863);
#8448=VERTEX_POINT('',#29864);
#8449=VERTEX_POINT('',#29866);
#8450=VERTEX_POINT('',#29868);
#8451=VERTEX_POINT('',#29872);
#8452=VERTEX_POINT('',#29873);
#8453=VERTEX_POINT('',#29875);
#8454=VERTEX_POINT('',#29877);
#8455=VERTEX_POINT('',#29881);
#8456=VERTEX_POINT('',#29882);
#8457=VERTEX_POINT('',#29884);
#8458=VERTEX_POINT('',#29886);
#8459=VERTEX_POINT('',#29890);
#8460=VERTEX_POINT('',#29891);
#8461=VERTEX_POINT('',#29893);
#8462=VERTEX_POINT('',#29895);
#8463=VERTEX_POINT('',#29899);
#8464=VERTEX_POINT('',#29900);
#8465=VERTEX_POINT('',#29902);
#8466=VERTEX_POINT('',#29904);
#8467=VERTEX_POINT('',#29908);
#8468=VERTEX_POINT('',#29909);
#8469=VERTEX_POINT('',#29911);
#8470=VERTEX_POINT('',#29913);
#8471=VERTEX_POINT('',#29917);
#8472=VERTEX_POINT('',#29918);
#8473=VERTEX_POINT('',#29920);
#8474=VERTEX_POINT('',#29922);
#8475=VERTEX_POINT('',#29926);
#8476=VERTEX_POINT('',#29927);
#8477=VERTEX_POINT('',#29929);
#8478=VERTEX_POINT('',#29931);
#8479=VERTEX_POINT('',#29935);
#8480=VERTEX_POINT('',#29936);
#8481=VERTEX_POINT('',#29938);
#8482=VERTEX_POINT('',#29940);
#8483=VERTEX_POINT('',#29944);
#8484=VERTEX_POINT('',#29945);
#8485=VERTEX_POINT('',#29947);
#8486=VERTEX_POINT('',#29949);
#8487=VERTEX_POINT('',#29953);
#8488=VERTEX_POINT('',#29954);
#8489=VERTEX_POINT('',#29956);
#8490=VERTEX_POINT('',#29958);
#8491=VERTEX_POINT('',#29962);
#8492=VERTEX_POINT('',#29963);
#8493=VERTEX_POINT('',#29965);
#8494=VERTEX_POINT('',#29967);
#8495=VERTEX_POINT('',#29971);
#8496=VERTEX_POINT('',#29972);
#8497=VERTEX_POINT('',#29974);
#8498=VERTEX_POINT('',#29976);
#8499=VERTEX_POINT('',#29980);
#8500=VERTEX_POINT('',#29981);
#8501=VERTEX_POINT('',#29983);
#8502=VERTEX_POINT('',#29985);
#8503=VERTEX_POINT('',#29989);
#8504=VERTEX_POINT('',#29990);
#8505=VERTEX_POINT('',#29992);
#8506=VERTEX_POINT('',#29994);
#8507=VERTEX_POINT('',#29998);
#8508=VERTEX_POINT('',#29999);
#8509=VERTEX_POINT('',#30001);
#8510=VERTEX_POINT('',#30003);
#8511=VERTEX_POINT('',#30007);
#8512=VERTEX_POINT('',#30008);
#8513=VERTEX_POINT('',#30010);
#8514=VERTEX_POINT('',#30012);
#8515=VERTEX_POINT('',#30016);
#8516=VERTEX_POINT('',#30017);
#8517=VERTEX_POINT('',#30019);
#8518=VERTEX_POINT('',#30021);
#8519=VERTEX_POINT('',#30025);
#8520=VERTEX_POINT('',#30026);
#8521=VERTEX_POINT('',#30028);
#8522=VERTEX_POINT('',#30030);
#8523=VERTEX_POINT('',#30034);
#8524=VERTEX_POINT('',#30035);
#8525=VERTEX_POINT('',#30037);
#8526=VERTEX_POINT('',#30039);
#8527=VERTEX_POINT('',#30043);
#8528=VERTEX_POINT('',#30044);
#8529=VERTEX_POINT('',#30046);
#8530=VERTEX_POINT('',#30048);
#8531=VERTEX_POINT('',#30052);
#8532=VERTEX_POINT('',#30053);
#8533=VERTEX_POINT('',#30055);
#8534=VERTEX_POINT('',#30057);
#8535=VERTEX_POINT('',#30061);
#8536=VERTEX_POINT('',#30062);
#8537=VERTEX_POINT('',#30064);
#8538=VERTEX_POINT('',#30066);
#8539=VERTEX_POINT('',#30070);
#8540=VERTEX_POINT('',#30071);
#8541=VERTEX_POINT('',#30073);
#8542=VERTEX_POINT('',#30075);
#8543=VERTEX_POINT('',#30079);
#8544=VERTEX_POINT('',#30080);
#8545=VERTEX_POINT('',#30082);
#8546=VERTEX_POINT('',#30084);
#8547=VERTEX_POINT('',#30088);
#8548=VERTEX_POINT('',#30089);
#8549=VERTEX_POINT('',#30091);
#8550=VERTEX_POINT('',#30093);
#8551=VERTEX_POINT('',#30097);
#8552=VERTEX_POINT('',#30098);
#8553=VERTEX_POINT('',#30100);
#8554=VERTEX_POINT('',#30102);
#8555=VERTEX_POINT('',#30106);
#8556=VERTEX_POINT('',#30107);
#8557=VERTEX_POINT('',#30109);
#8558=VERTEX_POINT('',#30111);
#8559=VERTEX_POINT('',#30115);
#8560=VERTEX_POINT('',#30116);
#8561=VERTEX_POINT('',#30118);
#8562=VERTEX_POINT('',#30120);
#8563=VERTEX_POINT('',#30124);
#8564=VERTEX_POINT('',#30125);
#8565=VERTEX_POINT('',#30127);
#8566=VERTEX_POINT('',#30129);
#8567=VERTEX_POINT('',#30133);
#8568=VERTEX_POINT('',#30134);
#8569=VERTEX_POINT('',#30136);
#8570=VERTEX_POINT('',#30138);
#8571=VERTEX_POINT('',#30142);
#8572=VERTEX_POINT('',#30143);
#8573=VERTEX_POINT('',#30145);
#8574=VERTEX_POINT('',#30147);
#8575=VERTEX_POINT('',#30151);
#8576=VERTEX_POINT('',#30153);
#8577=VERTEX_POINT('',#30199);
#8578=VERTEX_POINT('',#30202);
#8579=VERTEX_POINT('',#30206);
#8580=VERTEX_POINT('',#30297);
#10453=EDGE_CURVE('',#8399,#8400,#1387,.T.);
#10454=EDGE_CURVE('',#8401,#8399,#7101,.T.);
#10455=EDGE_CURVE('',#8402,#8401,#1388,.T.);
#10456=EDGE_CURVE('',#8400,#8402,#7102,.T.);
#10457=EDGE_CURVE('',#8403,#8404,#1389,.T.);
#10458=EDGE_CURVE('',#8405,#8403,#7103,.T.);
#10459=EDGE_CURVE('',#8406,#8405,#1390,.T.);
#10460=EDGE_CURVE('',#8404,#8406,#7104,.T.);
#10461=EDGE_CURVE('',#8407,#8408,#1391,.T.);
#10462=EDGE_CURVE('',#8409,#8407,#7105,.T.);
#10463=EDGE_CURVE('',#8410,#8409,#1392,.T.);
#10464=EDGE_CURVE('',#8408,#8410,#7106,.T.);
#10465=EDGE_CURVE('',#8411,#8412,#1393,.T.);
#10466=EDGE_CURVE('',#8413,#8411,#7107,.T.);
#10467=EDGE_CURVE('',#8414,#8413,#1394,.T.);
#10468=EDGE_CURVE('',#8412,#8414,#7108,.T.);
#10469=EDGE_CURVE('',#8415,#8416,#1395,.T.);
#10470=EDGE_CURVE('',#8417,#8415,#7109,.T.);
#10471=EDGE_CURVE('',#8418,#8417,#1396,.T.);
#10472=EDGE_CURVE('',#8416,#8418,#7110,.T.);
#10473=EDGE_CURVE('',#8419,#8420,#1397,.T.);
#10474=EDGE_CURVE('',#8421,#8419,#7111,.T.);
#10475=EDGE_CURVE('',#8422,#8421,#1398,.T.);
#10476=EDGE_CURVE('',#8420,#8422,#7112,.T.);
#10477=EDGE_CURVE('',#8423,#8424,#1399,.T.);
#10478=EDGE_CURVE('',#8425,#8423,#7113,.T.);
#10479=EDGE_CURVE('',#8426,#8425,#1400,.T.);
#10480=EDGE_CURVE('',#8424,#8426,#7114,.T.);
#10481=EDGE_CURVE('',#8427,#8428,#1401,.T.);
#10482=EDGE_CURVE('',#8429,#8427,#7115,.T.);
#10483=EDGE_CURVE('',#8430,#8429,#1402,.T.);
#10484=EDGE_CURVE('',#8428,#8430,#7116,.T.);
#10485=EDGE_CURVE('',#8431,#8432,#1403,.T.);
#10486=EDGE_CURVE('',#8433,#8431,#7117,.T.);
#10487=EDGE_CURVE('',#8434,#8433,#1404,.T.);
#10488=EDGE_CURVE('',#8432,#8434,#7118,.T.);
#10489=EDGE_CURVE('',#8435,#8436,#1405,.T.);
#10490=EDGE_CURVE('',#8437,#8435,#7119,.T.);
#10491=EDGE_CURVE('',#8438,#8437,#1406,.T.);
#10492=EDGE_CURVE('',#8436,#8438,#7120,.T.);
#10493=EDGE_CURVE('',#8439,#8440,#1407,.T.);
#10494=EDGE_CURVE('',#8441,#8439,#7121,.T.);
#10495=EDGE_CURVE('',#8442,#8441,#1408,.T.);
#10496=EDGE_CURVE('',#8440,#8442,#7122,.T.);
#10497=EDGE_CURVE('',#8443,#8444,#1409,.T.);
#10498=EDGE_CURVE('',#8445,#8443,#7123,.T.);
#10499=EDGE_CURVE('',#8446,#8445,#1410,.T.);
#10500=EDGE_CURVE('',#8444,#8446,#7124,.T.);
#10501=EDGE_CURVE('',#8447,#8448,#1411,.T.);
#10502=EDGE_CURVE('',#8449,#8447,#7125,.T.);
#10503=EDGE_CURVE('',#8450,#8449,#1412,.T.);
#10504=EDGE_CURVE('',#8448,#8450,#7126,.T.);
#10505=EDGE_CURVE('',#8451,#8452,#1413,.T.);
#10506=EDGE_CURVE('',#8453,#8451,#7127,.T.);
#10507=EDGE_CURVE('',#8454,#8453,#1414,.T.);
#10508=EDGE_CURVE('',#8452,#8454,#7128,.T.);
#10509=EDGE_CURVE('',#8455,#8456,#1415,.T.);
#10510=EDGE_CURVE('',#8457,#8455,#7129,.T.);
#10511=EDGE_CURVE('',#8458,#8457,#1416,.T.);
#10512=EDGE_CURVE('',#8456,#8458,#7130,.T.);
#10513=EDGE_CURVE('',#8459,#8460,#1417,.T.);
#10514=EDGE_CURVE('',#8461,#8459,#7131,.T.);
#10515=EDGE_CURVE('',#8462,#8461,#1418,.T.);
#10516=EDGE_CURVE('',#8460,#8462,#7132,.T.);
#10517=EDGE_CURVE('',#8463,#8464,#1419,.T.);
#10518=EDGE_CURVE('',#8465,#8463,#7133,.T.);
#10519=EDGE_CURVE('',#8466,#8465,#1420,.T.);
#10520=EDGE_CURVE('',#8464,#8466,#7134,.T.);
#10521=EDGE_CURVE('',#8467,#8468,#1421,.T.);
#10522=EDGE_CURVE('',#8469,#8467,#7135,.T.);
#10523=EDGE_CURVE('',#8470,#8469,#1422,.T.);
#10524=EDGE_CURVE('',#8468,#8470,#7136,.T.);
#10525=EDGE_CURVE('',#8471,#8472,#1423,.T.);
#10526=EDGE_CURVE('',#8473,#8471,#7137,.T.);
#10527=EDGE_CURVE('',#8474,#8473,#1424,.T.);
#10528=EDGE_CURVE('',#8472,#8474,#7138,.T.);
#10529=EDGE_CURVE('',#8475,#8476,#1425,.T.);
#10530=EDGE_CURVE('',#8477,#8475,#7139,.T.);
#10531=EDGE_CURVE('',#8478,#8477,#1426,.T.);
#10532=EDGE_CURVE('',#8476,#8478,#7140,.T.);
#10533=EDGE_CURVE('',#8479,#8480,#1427,.T.);
#10534=EDGE_CURVE('',#8481,#8479,#7141,.T.);
#10535=EDGE_CURVE('',#8482,#8481,#1428,.T.);
#10536=EDGE_CURVE('',#8480,#8482,#7142,.T.);
#10537=EDGE_CURVE('',#8483,#8484,#1429,.T.);
#10538=EDGE_CURVE('',#8485,#8483,#7143,.T.);
#10539=EDGE_CURVE('',#8486,#8485,#1430,.T.);
#10540=EDGE_CURVE('',#8484,#8486,#7144,.T.);
#10541=EDGE_CURVE('',#8487,#8488,#1431,.T.);
#10542=EDGE_CURVE('',#8489,#8487,#7145,.T.);
#10543=EDGE_CURVE('',#8490,#8489,#1432,.T.);
#10544=EDGE_CURVE('',#8488,#8490,#7146,.T.);
#10545=EDGE_CURVE('',#8491,#8492,#1433,.T.);
#10546=EDGE_CURVE('',#8493,#8491,#7147,.T.);
#10547=EDGE_CURVE('',#8494,#8493,#1434,.T.);
#10548=EDGE_CURVE('',#8492,#8494,#7148,.T.);
#10549=EDGE_CURVE('',#8495,#8496,#1435,.T.);
#10550=EDGE_CURVE('',#8497,#8495,#7149,.T.);
#10551=EDGE_CURVE('',#8498,#8497,#1436,.T.);
#10552=EDGE_CURVE('',#8496,#8498,#7150,.T.);
#10553=EDGE_CURVE('',#8499,#8500,#1437,.T.);
#10554=EDGE_CURVE('',#8501,#8499,#7151,.T.);
#10555=EDGE_CURVE('',#8502,#8501,#1438,.T.);
#10556=EDGE_CURVE('',#8500,#8502,#7152,.T.);
#10557=EDGE_CURVE('',#8503,#8504,#1439,.T.);
#10558=EDGE_CURVE('',#8505,#8503,#7153,.T.);
#10559=EDGE_CURVE('',#8506,#8505,#1440,.T.);
#10560=EDGE_CURVE('',#8504,#8506,#7154,.T.);
#10561=EDGE_CURVE('',#8507,#8508,#1441,.T.);
#10562=EDGE_CURVE('',#8509,#8507,#7155,.T.);
#10563=EDGE_CURVE('',#8510,#8509,#1442,.T.);
#10564=EDGE_CURVE('',#8508,#8510,#7156,.T.);
#10565=EDGE_CURVE('',#8511,#8512,#1443,.T.);
#10566=EDGE_CURVE('',#8513,#8511,#7157,.T.);
#10567=EDGE_CURVE('',#8514,#8513,#1444,.T.);
#10568=EDGE_CURVE('',#8512,#8514,#7158,.T.);
#10569=EDGE_CURVE('',#8515,#8516,#1445,.T.);
#10570=EDGE_CURVE('',#8517,#8515,#7159,.T.);
#10571=EDGE_CURVE('',#8518,#8517,#1446,.T.);
#10572=EDGE_CURVE('',#8516,#8518,#7160,.T.);
#10573=EDGE_CURVE('',#8519,#8520,#1447,.T.);
#10574=EDGE_CURVE('',#8521,#8519,#7161,.T.);
#10575=EDGE_CURVE('',#8522,#8521,#1448,.T.);
#10576=EDGE_CURVE('',#8520,#8522,#7162,.T.);
#10577=EDGE_CURVE('',#8523,#8524,#1449,.T.);
#10578=EDGE_CURVE('',#8525,#8523,#7163,.T.);
#10579=EDGE_CURVE('',#8526,#8525,#1450,.T.);
#10580=EDGE_CURVE('',#8524,#8526,#7164,.T.);
#10581=EDGE_CURVE('',#8527,#8528,#1451,.T.);
#10582=EDGE_CURVE('',#8529,#8527,#7165,.T.);
#10583=EDGE_CURVE('',#8530,#8529,#1452,.T.);
#10584=EDGE_CURVE('',#8528,#8530,#7166,.T.);
#10585=EDGE_CURVE('',#8531,#8532,#1453,.T.);
#10586=EDGE_CURVE('',#8533,#8531,#7167,.T.);
#10587=EDGE_CURVE('',#8534,#8533,#1454,.T.);
#10588=EDGE_CURVE('',#8532,#8534,#7168,.T.);
#10589=EDGE_CURVE('',#8535,#8536,#1455,.T.);
#10590=EDGE_CURVE('',#8537,#8535,#7169,.T.);
#10591=EDGE_CURVE('',#8538,#8537,#1456,.T.);
#10592=EDGE_CURVE('',#8536,#8538,#7170,.T.);
#10593=EDGE_CURVE('',#8539,#8540,#1457,.T.);
#10594=EDGE_CURVE('',#8541,#8539,#7171,.T.);
#10595=EDGE_CURVE('',#8542,#8541,#1458,.T.);
#10596=EDGE_CURVE('',#8540,#8542,#7172,.T.);
#10597=EDGE_CURVE('',#8543,#8544,#1459,.T.);
#10598=EDGE_CURVE('',#8545,#8543,#7173,.T.);
#10599=EDGE_CURVE('',#8546,#8545,#1460,.T.);
#10600=EDGE_CURVE('',#8544,#8546,#7174,.T.);
#10601=EDGE_CURVE('',#8547,#8548,#1461,.T.);
#10602=EDGE_CURVE('',#8549,#8547,#7175,.T.);
#10603=EDGE_CURVE('',#8550,#8549,#1462,.T.);
#10604=EDGE_CURVE('',#8548,#8550,#7176,.T.);
#10605=EDGE_CURVE('',#8551,#8552,#1463,.T.);
#10606=EDGE_CURVE('',#8553,#8551,#7177,.T.);
#10607=EDGE_CURVE('',#8554,#8553,#1464,.T.);
#10608=EDGE_CURVE('',#8552,#8554,#7178,.T.);
#10609=EDGE_CURVE('',#8555,#8556,#1465,.T.);
#10610=EDGE_CURVE('',#8557,#8555,#7179,.T.);
#10611=EDGE_CURVE('',#8558,#8557,#1466,.T.);
#10612=EDGE_CURVE('',#8556,#8558,#7180,.T.);
#10613=EDGE_CURVE('',#8559,#8560,#1467,.T.);
#10614=EDGE_CURVE('',#8561,#8559,#7181,.T.);
#10615=EDGE_CURVE('',#8562,#8561,#1468,.T.);
#10616=EDGE_CURVE('',#8560,#8562,#7182,.T.);
#10617=EDGE_CURVE('',#8563,#8564,#1469,.T.);
#10618=EDGE_CURVE('',#8565,#8563,#7183,.T.);
#10619=EDGE_CURVE('',#8566,#8565,#1470,.T.);
#10620=EDGE_CURVE('',#8564,#8566,#7184,.T.);
#10621=EDGE_CURVE('',#8567,#8568,#1471,.T.);
#10622=EDGE_CURVE('',#8569,#8567,#7185,.T.);
#10623=EDGE_CURVE('',#8570,#8569,#1472,.T.);
#10624=EDGE_CURVE('',#8568,#8570,#7186,.T.);
#10625=EDGE_CURVE('',#8571,#8572,#1473,.T.);
#10626=EDGE_CURVE('',#8573,#8571,#7187,.T.);
#10627=EDGE_CURVE('',#8574,#8573,#1474,.T.);
#10628=EDGE_CURVE('',#8572,#8574,#7188,.T.);
#10629=EDGE_CURVE('',#8402,#8575,#7189,.T.);
#10630=EDGE_CURVE('',#8575,#8576,#7190,.T.);
#10631=EDGE_CURVE('',#8576,#8572,#7191,.T.);
#10632=EDGE_CURVE('',#8574,#8568,#7192,.T.);
#10633=EDGE_CURVE('',#8570,#8564,#7193,.T.);
#10634=EDGE_CURVE('',#8566,#8560,#7194,.T.);
#10635=EDGE_CURVE('',#8562,#8556,#7195,.T.);
#10636=EDGE_CURVE('',#8558,#8552,#7196,.T.);
#10637=EDGE_CURVE('',#8554,#8548,#7197,.T.);
#10638=EDGE_CURVE('',#8550,#8544,#7198,.T.);
#10639=EDGE_CURVE('',#8546,#8540,#7199,.T.);
#10640=EDGE_CURVE('',#8542,#8536,#7200,.T.);
#10641=EDGE_CURVE('',#8538,#8532,#7201,.T.);
#10642=EDGE_CURVE('',#8534,#8528,#7202,.T.);
#10643=EDGE_CURVE('',#8530,#8524,#7203,.T.);
#10644=EDGE_CURVE('',#8526,#8520,#7204,.T.);
#10645=EDGE_CURVE('',#8522,#8516,#7205,.T.);
#10646=EDGE_CURVE('',#8518,#8512,#7206,.T.);
#10647=EDGE_CURVE('',#8514,#8508,#7207,.T.);
#10648=EDGE_CURVE('',#8510,#8504,#7208,.T.);
#10649=EDGE_CURVE('',#8506,#8500,#7209,.T.);
#10650=EDGE_CURVE('',#8502,#8496,#7210,.T.);
#10651=EDGE_CURVE('',#8498,#8492,#7211,.T.);
#10652=EDGE_CURVE('',#8494,#8488,#7212,.T.);
#10653=EDGE_CURVE('',#8490,#8484,#7213,.T.);
#10654=EDGE_CURVE('',#8486,#8480,#7214,.T.);
#10655=EDGE_CURVE('',#8482,#8476,#7215,.T.);
#10656=EDGE_CURVE('',#8478,#8472,#7216,.T.);
#10657=EDGE_CURVE('',#8474,#8468,#7217,.T.);
#10658=EDGE_CURVE('',#8470,#8464,#7218,.T.);
#10659=EDGE_CURVE('',#8466,#8460,#7219,.T.);
#10660=EDGE_CURVE('',#8462,#8456,#7220,.T.);
#10661=EDGE_CURVE('',#8458,#8452,#7221,.T.);
#10662=EDGE_CURVE('',#8454,#8448,#7222,.T.);
#10663=EDGE_CURVE('',#8450,#8444,#7223,.T.);
#10664=EDGE_CURVE('',#8446,#8440,#7224,.T.);
#10665=EDGE_CURVE('',#8442,#8436,#7225,.T.);
#10666=EDGE_CURVE('',#8438,#8432,#7226,.T.);
#10667=EDGE_CURVE('',#8434,#8428,#7227,.T.);
#10668=EDGE_CURVE('',#8430,#8424,#7228,.T.);
#10669=EDGE_CURVE('',#8426,#8420,#7229,.T.);
#10670=EDGE_CURVE('',#8422,#8416,#7230,.T.);
#10671=EDGE_CURVE('',#8418,#8412,#7231,.T.);
#10672=EDGE_CURVE('',#8414,#8408,#7232,.T.);
#10673=EDGE_CURVE('',#8410,#8404,#7233,.T.);
#10674=EDGE_CURVE('',#8406,#8400,#7234,.T.);
#10675=EDGE_CURVE('',#8577,#8577,#7235,.T.);
#10676=EDGE_CURVE('',#8578,#8401,#7236,.T.);
#10677=EDGE_CURVE('',#8578,#8575,#1475,.T.);
#10678=EDGE_CURVE('',#8576,#8579,#1476,.T.);
#10679=EDGE_CURVE('',#8571,#8579,#7237,.T.);
#10680=EDGE_CURVE('',#8567,#8573,#7238,.T.);
#10681=EDGE_CURVE('',#8563,#8569,#7239,.T.);
#10682=EDGE_CURVE('',#8559,#8565,#7240,.T.);
#10683=EDGE_CURVE('',#8555,#8561,#7241,.T.);
#10684=EDGE_CURVE('',#8551,#8557,#7242,.T.);
#10685=EDGE_CURVE('',#8547,#8553,#7243,.T.);
#10686=EDGE_CURVE('',#8543,#8549,#7244,.T.);
#10687=EDGE_CURVE('',#8539,#8545,#7245,.T.);
#10688=EDGE_CURVE('',#8535,#8541,#7246,.T.);
#10689=EDGE_CURVE('',#8531,#8537,#7247,.T.);
#10690=EDGE_CURVE('',#8527,#8533,#7248,.T.);
#10691=EDGE_CURVE('',#8523,#8529,#7249,.T.);
#10692=EDGE_CURVE('',#8519,#8525,#7250,.T.);
#10693=EDGE_CURVE('',#8515,#8521,#7251,.T.);
#10694=EDGE_CURVE('',#8511,#8517,#7252,.T.);
#10695=EDGE_CURVE('',#8507,#8513,#7253,.T.);
#10696=EDGE_CURVE('',#8503,#8509,#7254,.T.);
#10697=EDGE_CURVE('',#8499,#8505,#7255,.T.);
#10698=EDGE_CURVE('',#8495,#8501,#7256,.T.);
#10699=EDGE_CURVE('',#8491,#8497,#7257,.T.);
#10700=EDGE_CURVE('',#8487,#8493,#7258,.T.);
#10701=EDGE_CURVE('',#8483,#8489,#7259,.T.);
#10702=EDGE_CURVE('',#8479,#8485,#7260,.T.);
#10703=EDGE_CURVE('',#8475,#8481,#7261,.T.);
#10704=EDGE_CURVE('',#8471,#8477,#7262,.T.);
#10705=EDGE_CURVE('',#8467,#8473,#7263,.T.);
#10706=EDGE_CURVE('',#8463,#8469,#7264,.T.);
#10707=EDGE_CURVE('',#8459,#8465,#7265,.T.);
#10708=EDGE_CURVE('',#8455,#8461,#7266,.T.);
#10709=EDGE_CURVE('',#8451,#8457,#7267,.T.);
#10710=EDGE_CURVE('',#8447,#8453,#7268,.T.);
#10711=EDGE_CURVE('',#8443,#8449,#7269,.T.);
#10712=EDGE_CURVE('',#8439,#8445,#7270,.T.);
#10713=EDGE_CURVE('',#8435,#8441,#7271,.T.);
#10714=EDGE_CURVE('',#8431,#8437,#7272,.T.);
#10715=EDGE_CURVE('',#8427,#8433,#7273,.T.);
#10716=EDGE_CURVE('',#8423,#8429,#7274,.T.);
#10717=EDGE_CURVE('',#8419,#8425,#7275,.T.);
#10718=EDGE_CURVE('',#8415,#8421,#7276,.T.);
#10719=EDGE_CURVE('',#8411,#8417,#7277,.T.);
#10720=EDGE_CURVE('',#8407,#8413,#7278,.T.);
#10721=EDGE_CURVE('',#8403,#8409,#7279,.T.);
#10722=EDGE_CURVE('',#8579,#8578,#7280,.T.);
#10723=EDGE_CURVE('',#8399,#8405,#7281,.T.);
#10724=EDGE_CURVE('',#8580,#8580,#7282,.T.);
#10725=EDGE_CURVE('',#8580,#8577,#1477,.T.);
#13790=ORIENTED_EDGE('',*,*,#10453,.F.);
#13791=ORIENTED_EDGE('',*,*,#10454,.F.);
#13792=ORIENTED_EDGE('',*,*,#10455,.F.);
#13793=ORIENTED_EDGE('',*,*,#10456,.F.);
#13794=ORIENTED_EDGE('',*,*,#10457,.F.);
#13795=ORIENTED_EDGE('',*,*,#10458,.F.);
#13796=ORIENTED_EDGE('',*,*,#10459,.F.);
#13797=ORIENTED_EDGE('',*,*,#10460,.F.);
#13798=ORIENTED_EDGE('',*,*,#10461,.F.);
#13799=ORIENTED_EDGE('',*,*,#10462,.F.);
#13800=ORIENTED_EDGE('',*,*,#10463,.F.);
#13801=ORIENTED_EDGE('',*,*,#10464,.F.);
#13802=ORIENTED_EDGE('',*,*,#10465,.F.);
#13803=ORIENTED_EDGE('',*,*,#10466,.F.);
#13804=ORIENTED_EDGE('',*,*,#10467,.F.);
#13805=ORIENTED_EDGE('',*,*,#10468,.F.);
#13806=ORIENTED_EDGE('',*,*,#10469,.F.);
#13807=ORIENTED_EDGE('',*,*,#10470,.F.);
#13808=ORIENTED_EDGE('',*,*,#10471,.F.);
#13809=ORIENTED_EDGE('',*,*,#10472,.F.);
#13810=ORIENTED_EDGE('',*,*,#10473,.F.);
#13811=ORIENTED_EDGE('',*,*,#10474,.F.);
#13812=ORIENTED_EDGE('',*,*,#10475,.F.);
#13813=ORIENTED_EDGE('',*,*,#10476,.F.);
#13814=ORIENTED_EDGE('',*,*,#10477,.F.);
#13815=ORIENTED_EDGE('',*,*,#10478,.F.);
#13816=ORIENTED_EDGE('',*,*,#10479,.F.);
#13817=ORIENTED_EDGE('',*,*,#10480,.F.);
#13818=ORIENTED_EDGE('',*,*,#10481,.F.);
#13819=ORIENTED_EDGE('',*,*,#10482,.F.);
#13820=ORIENTED_EDGE('',*,*,#10483,.F.);
#13821=ORIENTED_EDGE('',*,*,#10484,.F.);
#13822=ORIENTED_EDGE('',*,*,#10485,.F.);
#13823=ORIENTED_EDGE('',*,*,#10486,.F.);
#13824=ORIENTED_EDGE('',*,*,#10487,.F.);
#13825=ORIENTED_EDGE('',*,*,#10488,.F.);
#13826=ORIENTED_EDGE('',*,*,#10489,.F.);
#13827=ORIENTED_EDGE('',*,*,#10490,.F.);
#13828=ORIENTED_EDGE('',*,*,#10491,.F.);
#13829=ORIENTED_EDGE('',*,*,#10492,.F.);
#13830=ORIENTED_EDGE('',*,*,#10493,.F.);
#13831=ORIENTED_EDGE('',*,*,#10494,.F.);
#13832=ORIENTED_EDGE('',*,*,#10495,.F.);
#13833=ORIENTED_EDGE('',*,*,#10496,.F.);
#13834=ORIENTED_EDGE('',*,*,#10497,.F.);
#13835=ORIENTED_EDGE('',*,*,#10498,.F.);
#13836=ORIENTED_EDGE('',*,*,#10499,.F.);
#13837=ORIENTED_EDGE('',*,*,#10500,.F.);
#13838=ORIENTED_EDGE('',*,*,#10501,.F.);
#13839=ORIENTED_EDGE('',*,*,#10502,.F.);
#13840=ORIENTED_EDGE('',*,*,#10503,.F.);
#13841=ORIENTED_EDGE('',*,*,#10504,.F.);
#13842=ORIENTED_EDGE('',*,*,#10505,.F.);
#13843=ORIENTED_EDGE('',*,*,#10506,.F.);
#13844=ORIENTED_EDGE('',*,*,#10507,.F.);
#13845=ORIENTED_EDGE('',*,*,#10508,.F.);
#13846=ORIENTED_EDGE('',*,*,#10509,.F.);
#13847=ORIENTED_EDGE('',*,*,#10510,.F.);
#13848=ORIENTED_EDGE('',*,*,#10511,.F.);
#13849=ORIENTED_EDGE('',*,*,#10512,.F.);
#13850=ORIENTED_EDGE('',*,*,#10513,.F.);
#13851=ORIENTED_EDGE('',*,*,#10514,.F.);
#13852=ORIENTED_EDGE('',*,*,#10515,.F.);
#13853=ORIENTED_EDGE('',*,*,#10516,.F.);
#13854=ORIENTED_EDGE('',*,*,#10517,.F.);
#13855=ORIENTED_EDGE('',*,*,#10518,.F.);
#13856=ORIENTED_EDGE('',*,*,#10519,.F.);
#13857=ORIENTED_EDGE('',*,*,#10520,.F.);
#13858=ORIENTED_EDGE('',*,*,#10521,.F.);
#13859=ORIENTED_EDGE('',*,*,#10522,.F.);
#13860=ORIENTED_EDGE('',*,*,#10523,.F.);
#13861=ORIENTED_EDGE('',*,*,#10524,.F.);
#13862=ORIENTED_EDGE('',*,*,#10525,.F.);
#13863=ORIENTED_EDGE('',*,*,#10526,.F.);
#13864=ORIENTED_EDGE('',*,*,#10527,.F.);
#13865=ORIENTED_EDGE('',*,*,#10528,.F.);
#13866=ORIENTED_EDGE('',*,*,#10529,.F.);
#13867=ORIENTED_EDGE('',*,*,#10530,.F.);
#13868=ORIENTED_EDGE('',*,*,#10531,.F.);
#13869=ORIENTED_EDGE('',*,*,#10532,.F.);
#13870=ORIENTED_EDGE('',*,*,#10533,.F.);
#13871=ORIENTED_EDGE('',*,*,#10534,.F.);
#13872=ORIENTED_EDGE('',*,*,#10535,.F.);
#13873=ORIENTED_EDGE('',*,*,#10536,.F.);
#13874=ORIENTED_EDGE('',*,*,#10537,.F.);
#13875=ORIENTED_EDGE('',*,*,#10538,.F.);
#13876=ORIENTED_EDGE('',*,*,#10539,.F.);
#13877=ORIENTED_EDGE('',*,*,#10540,.F.);
#13878=ORIENTED_EDGE('',*,*,#10541,.F.);
#13879=ORIENTED_EDGE('',*,*,#10542,.F.);
#13880=ORIENTED_EDGE('',*,*,#10543,.F.);
#13881=ORIENTED_EDGE('',*,*,#10544,.F.);
#13882=ORIENTED_EDGE('',*,*,#10545,.F.);
#13883=ORIENTED_EDGE('',*,*,#10546,.F.);
#13884=ORIENTED_EDGE('',*,*,#10547,.F.);
#13885=ORIENTED_EDGE('',*,*,#10548,.F.);
#13886=ORIENTED_EDGE('',*,*,#10549,.F.);
#13887=ORIENTED_EDGE('',*,*,#10550,.F.);
#13888=ORIENTED_EDGE('',*,*,#10551,.F.);
#13889=ORIENTED_EDGE('',*,*,#10552,.F.);
#13890=ORIENTED_EDGE('',*,*,#10553,.F.);
#13891=ORIENTED_EDGE('',*,*,#10554,.F.);
#13892=ORIENTED_EDGE('',*,*,#10555,.F.);
#13893=ORIENTED_EDGE('',*,*,#10556,.F.);
#13894=ORIENTED_EDGE('',*,*,#10557,.F.);
#13895=ORIENTED_EDGE('',*,*,#10558,.F.);
#13896=ORIENTED_EDGE('',*,*,#10559,.F.);
#13897=ORIENTED_EDGE('',*,*,#10560,.F.);
#13898=ORIENTED_EDGE('',*,*,#10561,.F.);
#13899=ORIENTED_EDGE('',*,*,#10562,.F.);
#13900=ORIENTED_EDGE('',*,*,#10563,.F.);
#13901=ORIENTED_EDGE('',*,*,#10564,.F.);
#13902=ORIENTED_EDGE('',*,*,#10565,.F.);
#13903=ORIENTED_EDGE('',*,*,#10566,.F.);
#13904=ORIENTED_EDGE('',*,*,#10567,.F.);
#13905=ORIENTED_EDGE('',*,*,#10568,.F.);
#13906=ORIENTED_EDGE('',*,*,#10569,.F.);
#13907=ORIENTED_EDGE('',*,*,#10570,.F.);
#13908=ORIENTED_EDGE('',*,*,#10571,.F.);
#13909=ORIENTED_EDGE('',*,*,#10572,.F.);
#13910=ORIENTED_EDGE('',*,*,#10573,.F.);
#13911=ORIENTED_EDGE('',*,*,#10574,.F.);
#13912=ORIENTED_EDGE('',*,*,#10575,.F.);
#13913=ORIENTED_EDGE('',*,*,#10576,.F.);
#13914=ORIENTED_EDGE('',*,*,#10577,.F.);
#13915=ORIENTED_EDGE('',*,*,#10578,.F.);
#13916=ORIENTED_EDGE('',*,*,#10579,.F.);
#13917=ORIENTED_EDGE('',*,*,#10580,.F.);
#13918=ORIENTED_EDGE('',*,*,#10581,.F.);
#13919=ORIENTED_EDGE('',*,*,#10582,.F.);
#13920=ORIENTED_EDGE('',*,*,#10583,.F.);
#13921=ORIENTED_EDGE('',*,*,#10584,.F.);
#13922=ORIENTED_EDGE('',*,*,#10585,.F.);
#13923=ORIENTED_EDGE('',*,*,#10586,.F.);
#13924=ORIENTED_EDGE('',*,*,#10587,.F.);
#13925=ORIENTED_EDGE('',*,*,#10588,.F.);
#13926=ORIENTED_EDGE('',*,*,#10589,.F.);
#13927=ORIENTED_EDGE('',*,*,#10590,.F.);
#13928=ORIENTED_EDGE('',*,*,#10591,.F.);
#13929=ORIENTED_EDGE('',*,*,#10592,.F.);
#13930=ORIENTED_EDGE('',*,*,#10593,.F.);
#13931=ORIENTED_EDGE('',*,*,#10594,.F.);
#13932=ORIENTED_EDGE('',*,*,#10595,.F.);
#13933=ORIENTED_EDGE('',*,*,#10596,.F.);
#13934=ORIENTED_EDGE('',*,*,#10597,.F.);
#13935=ORIENTED_EDGE('',*,*,#10598,.F.);
#13936=ORIENTED_EDGE('',*,*,#10599,.F.);
#13937=ORIENTED_EDGE('',*,*,#10600,.F.);
#13938=ORIENTED_EDGE('',*,*,#10601,.F.);
#13939=ORIENTED_EDGE('',*,*,#10602,.F.);
#13940=ORIENTED_EDGE('',*,*,#10603,.F.);
#13941=ORIENTED_EDGE('',*,*,#10604,.F.);
#13942=ORIENTED_EDGE('',*,*,#10605,.F.);
#13943=ORIENTED_EDGE('',*,*,#10606,.F.);
#13944=ORIENTED_EDGE('',*,*,#10607,.F.);
#13945=ORIENTED_EDGE('',*,*,#10608,.F.);
#13946=ORIENTED_EDGE('',*,*,#10609,.F.);
#13947=ORIENTED_EDGE('',*,*,#10610,.F.);
#13948=ORIENTED_EDGE('',*,*,#10611,.F.);
#13949=ORIENTED_EDGE('',*,*,#10612,.F.);
#13950=ORIENTED_EDGE('',*,*,#10613,.F.);
#13951=ORIENTED_EDGE('',*,*,#10614,.F.);
#13952=ORIENTED_EDGE('',*,*,#10615,.F.);
#13953=ORIENTED_EDGE('',*,*,#10616,.F.);
#13954=ORIENTED_EDGE('',*,*,#10617,.F.);
#13955=ORIENTED_EDGE('',*,*,#10618,.F.);
#13956=ORIENTED_EDGE('',*,*,#10619,.F.);
#13957=ORIENTED_EDGE('',*,*,#10620,.F.);
#13958=ORIENTED_EDGE('',*,*,#10621,.F.);
#13959=ORIENTED_EDGE('',*,*,#10622,.F.);
#13960=ORIENTED_EDGE('',*,*,#10623,.F.);
#13961=ORIENTED_EDGE('',*,*,#10624,.F.);
#13962=ORIENTED_EDGE('',*,*,#10625,.F.);
#13963=ORIENTED_EDGE('',*,*,#10626,.F.);
#13964=ORIENTED_EDGE('',*,*,#10627,.F.);
#13965=ORIENTED_EDGE('',*,*,#10628,.F.);
#13966=ORIENTED_EDGE('',*,*,#10456,.T.);
#13967=ORIENTED_EDGE('',*,*,#10629,.T.);
#13968=ORIENTED_EDGE('',*,*,#10630,.T.);
#13969=ORIENTED_EDGE('',*,*,#10631,.T.);
#13970=ORIENTED_EDGE('',*,*,#10628,.T.);
#13971=ORIENTED_EDGE('',*,*,#10632,.T.);
#13972=ORIENTED_EDGE('',*,*,#10624,.T.);
#13973=ORIENTED_EDGE('',*,*,#10633,.T.);
#13974=ORIENTED_EDGE('',*,*,#10620,.T.);
#13975=ORIENTED_EDGE('',*,*,#10634,.T.);
#13976=ORIENTED_EDGE('',*,*,#10616,.T.);
#13977=ORIENTED_EDGE('',*,*,#10635,.T.);
#13978=ORIENTED_EDGE('',*,*,#10612,.T.);
#13979=ORIENTED_EDGE('',*,*,#10636,.T.);
#13980=ORIENTED_EDGE('',*,*,#10608,.T.);
#13981=ORIENTED_EDGE('',*,*,#10637,.T.);
#13982=ORIENTED_EDGE('',*,*,#10604,.T.);
#13983=ORIENTED_EDGE('',*,*,#10638,.T.);
#13984=ORIENTED_EDGE('',*,*,#10600,.T.);
#13985=ORIENTED_EDGE('',*,*,#10639,.T.);
#13986=ORIENTED_EDGE('',*,*,#10596,.T.);
#13987=ORIENTED_EDGE('',*,*,#10640,.T.);
#13988=ORIENTED_EDGE('',*,*,#10592,.T.);
#13989=ORIENTED_EDGE('',*,*,#10641,.T.);
#13990=ORIENTED_EDGE('',*,*,#10588,.T.);
#13991=ORIENTED_EDGE('',*,*,#10642,.T.);
#13992=ORIENTED_EDGE('',*,*,#10584,.T.);
#13993=ORIENTED_EDGE('',*,*,#10643,.T.);
#13994=ORIENTED_EDGE('',*,*,#10580,.T.);
#13995=ORIENTED_EDGE('',*,*,#10644,.T.);
#13996=ORIENTED_EDGE('',*,*,#10576,.T.);
#13997=ORIENTED_EDGE('',*,*,#10645,.T.);
#13998=ORIENTED_EDGE('',*,*,#10572,.T.);
#13999=ORIENTED_EDGE('',*,*,#10646,.T.);
#14000=ORIENTED_EDGE('',*,*,#10568,.T.);
#14001=ORIENTED_EDGE('',*,*,#10647,.T.);
#14002=ORIENTED_EDGE('',*,*,#10564,.T.);
#14003=ORIENTED_EDGE('',*,*,#10648,.T.);
#14004=ORIENTED_EDGE('',*,*,#10560,.T.);
#14005=ORIENTED_EDGE('',*,*,#10649,.T.);
#14006=ORIENTED_EDGE('',*,*,#10556,.T.);
#14007=ORIENTED_EDGE('',*,*,#10650,.T.);
#14008=ORIENTED_EDGE('',*,*,#10552,.T.);
#14009=ORIENTED_EDGE('',*,*,#10651,.T.);
#14010=ORIENTED_EDGE('',*,*,#10548,.T.);
#14011=ORIENTED_EDGE('',*,*,#10652,.T.);
#14012=ORIENTED_EDGE('',*,*,#10544,.T.);
#14013=ORIENTED_EDGE('',*,*,#10653,.T.);
#14014=ORIENTED_EDGE('',*,*,#10540,.T.);
#14015=ORIENTED_EDGE('',*,*,#10654,.T.);
#14016=ORIENTED_EDGE('',*,*,#10536,.T.);
#14017=ORIENTED_EDGE('',*,*,#10655,.T.);
#14018=ORIENTED_EDGE('',*,*,#10532,.T.);
#14019=ORIENTED_EDGE('',*,*,#10656,.T.);
#14020=ORIENTED_EDGE('',*,*,#10528,.T.);
#14021=ORIENTED_EDGE('',*,*,#10657,.T.);
#14022=ORIENTED_EDGE('',*,*,#10524,.T.);
#14023=ORIENTED_EDGE('',*,*,#10658,.T.);
#14024=ORIENTED_EDGE('',*,*,#10520,.T.);
#14025=ORIENTED_EDGE('',*,*,#10659,.T.);
#14026=ORIENTED_EDGE('',*,*,#10516,.T.);
#14027=ORIENTED_EDGE('',*,*,#10660,.T.);
#14028=ORIENTED_EDGE('',*,*,#10512,.T.);
#14029=ORIENTED_EDGE('',*,*,#10661,.T.);
#14030=ORIENTED_EDGE('',*,*,#10508,.T.);
#14031=ORIENTED_EDGE('',*,*,#10662,.T.);
#14032=ORIENTED_EDGE('',*,*,#10504,.T.);
#14033=ORIENTED_EDGE('',*,*,#10663,.T.);
#14034=ORIENTED_EDGE('',*,*,#10500,.T.);
#14035=ORIENTED_EDGE('',*,*,#10664,.T.);
#14036=ORIENTED_EDGE('',*,*,#10496,.T.);
#14037=ORIENTED_EDGE('',*,*,#10665,.T.);
#14038=ORIENTED_EDGE('',*,*,#10492,.T.);
#14039=ORIENTED_EDGE('',*,*,#10666,.T.);
#14040=ORIENTED_EDGE('',*,*,#10488,.T.);
#14041=ORIENTED_EDGE('',*,*,#10667,.T.);
#14042=ORIENTED_EDGE('',*,*,#10484,.T.);
#14043=ORIENTED_EDGE('',*,*,#10668,.T.);
#14044=ORIENTED_EDGE('',*,*,#10480,.T.);
#14045=ORIENTED_EDGE('',*,*,#10669,.T.);
#14046=ORIENTED_EDGE('',*,*,#10476,.T.);
#14047=ORIENTED_EDGE('',*,*,#10670,.T.);
#14048=ORIENTED_EDGE('',*,*,#10472,.T.);
#14049=ORIENTED_EDGE('',*,*,#10671,.T.);
#14050=ORIENTED_EDGE('',*,*,#10468,.T.);
#14051=ORIENTED_EDGE('',*,*,#10672,.T.);
#14052=ORIENTED_EDGE('',*,*,#10464,.T.);
#14053=ORIENTED_EDGE('',*,*,#10673,.T.);
#14054=ORIENTED_EDGE('',*,*,#10460,.T.);
#14055=ORIENTED_EDGE('',*,*,#10674,.T.);
#14056=ORIENTED_EDGE('',*,*,#10675,.T.);
#14057=ORIENTED_EDGE('',*,*,#10455,.T.);
#14058=ORIENTED_EDGE('',*,*,#10676,.F.);
#14059=ORIENTED_EDGE('',*,*,#10677,.T.);
#14060=ORIENTED_EDGE('',*,*,#10629,.F.);
#14061=ORIENTED_EDGE('',*,*,#10625,.T.);
#14062=ORIENTED_EDGE('',*,*,#10631,.F.);
#14063=ORIENTED_EDGE('',*,*,#10678,.T.);
#14064=ORIENTED_EDGE('',*,*,#10679,.F.);
#14065=ORIENTED_EDGE('',*,*,#10621,.T.);
#14066=ORIENTED_EDGE('',*,*,#10632,.F.);
#14067=ORIENTED_EDGE('',*,*,#10627,.T.);
#14068=ORIENTED_EDGE('',*,*,#10680,.F.);
#14069=ORIENTED_EDGE('',*,*,#10617,.T.);
#14070=ORIENTED_EDGE('',*,*,#10633,.F.);
#14071=ORIENTED_EDGE('',*,*,#10623,.T.);
#14072=ORIENTED_EDGE('',*,*,#10681,.F.);
#14073=ORIENTED_EDGE('',*,*,#10613,.T.);
#14074=ORIENTED_EDGE('',*,*,#10634,.F.);
#14075=ORIENTED_EDGE('',*,*,#10619,.T.);
#14076=ORIENTED_EDGE('',*,*,#10682,.F.);
#14077=ORIENTED_EDGE('',*,*,#10609,.T.);
#14078=ORIENTED_EDGE('',*,*,#10635,.F.);
#14079=ORIENTED_EDGE('',*,*,#10615,.T.);
#14080=ORIENTED_EDGE('',*,*,#10683,.F.);
#14081=ORIENTED_EDGE('',*,*,#10605,.T.);
#14082=ORIENTED_EDGE('',*,*,#10636,.F.);
#14083=ORIENTED_EDGE('',*,*,#10611,.T.);
#14084=ORIENTED_EDGE('',*,*,#10684,.F.);
#14085=ORIENTED_EDGE('',*,*,#10601,.T.);
#14086=ORIENTED_EDGE('',*,*,#10637,.F.);
#14087=ORIENTED_EDGE('',*,*,#10607,.T.);
#14088=ORIENTED_EDGE('',*,*,#10685,.F.);
#14089=ORIENTED_EDGE('',*,*,#10597,.T.);
#14090=ORIENTED_EDGE('',*,*,#10638,.F.);
#14091=ORIENTED_EDGE('',*,*,#10603,.T.);
#14092=ORIENTED_EDGE('',*,*,#10686,.F.);
#14093=ORIENTED_EDGE('',*,*,#10593,.T.);
#14094=ORIENTED_EDGE('',*,*,#10639,.F.);
#14095=ORIENTED_EDGE('',*,*,#10599,.T.);
#14096=ORIENTED_EDGE('',*,*,#10687,.F.);
#14097=ORIENTED_EDGE('',*,*,#10589,.T.);
#14098=ORIENTED_EDGE('',*,*,#10640,.F.);
#14099=ORIENTED_EDGE('',*,*,#10595,.T.);
#14100=ORIENTED_EDGE('',*,*,#10688,.F.);
#14101=ORIENTED_EDGE('',*,*,#10585,.T.);
#14102=ORIENTED_EDGE('',*,*,#10641,.F.);
#14103=ORIENTED_EDGE('',*,*,#10591,.T.);
#14104=ORIENTED_EDGE('',*,*,#10689,.F.);
#14105=ORIENTED_EDGE('',*,*,#10581,.T.);
#14106=ORIENTED_EDGE('',*,*,#10642,.F.);
#14107=ORIENTED_EDGE('',*,*,#10587,.T.);
#14108=ORIENTED_EDGE('',*,*,#10690,.F.);
#14109=ORIENTED_EDGE('',*,*,#10577,.T.);
#14110=ORIENTED_EDGE('',*,*,#10643,.F.);
#14111=ORIENTED_EDGE('',*,*,#10583,.T.);
#14112=ORIENTED_EDGE('',*,*,#10691,.F.);
#14113=ORIENTED_EDGE('',*,*,#10573,.T.);
#14114=ORIENTED_EDGE('',*,*,#10644,.F.);
#14115=ORIENTED_EDGE('',*,*,#10579,.T.);
#14116=ORIENTED_EDGE('',*,*,#10692,.F.);
#14117=ORIENTED_EDGE('',*,*,#10569,.T.);
#14118=ORIENTED_EDGE('',*,*,#10645,.F.);
#14119=ORIENTED_EDGE('',*,*,#10575,.T.);
#14120=ORIENTED_EDGE('',*,*,#10693,.F.);
#14121=ORIENTED_EDGE('',*,*,#10565,.T.);
#14122=ORIENTED_EDGE('',*,*,#10646,.F.);
#14123=ORIENTED_EDGE('',*,*,#10571,.T.);
#14124=ORIENTED_EDGE('',*,*,#10694,.F.);
#14125=ORIENTED_EDGE('',*,*,#10561,.T.);
#14126=ORIENTED_EDGE('',*,*,#10647,.F.);
#14127=ORIENTED_EDGE('',*,*,#10567,.T.);
#14128=ORIENTED_EDGE('',*,*,#10695,.F.);
#14129=ORIENTED_EDGE('',*,*,#10557,.T.);
#14130=ORIENTED_EDGE('',*,*,#10648,.F.);
#14131=ORIENTED_EDGE('',*,*,#10563,.T.);
#14132=ORIENTED_EDGE('',*,*,#10696,.F.);
#14133=ORIENTED_EDGE('',*,*,#10553,.T.);
#14134=ORIENTED_EDGE('',*,*,#10649,.F.);
#14135=ORIENTED_EDGE('',*,*,#10559,.T.);
#14136=ORIENTED_EDGE('',*,*,#10697,.F.);
#14137=ORIENTED_EDGE('',*,*,#10549,.T.);
#14138=ORIENTED_EDGE('',*,*,#10650,.F.);
#14139=ORIENTED_EDGE('',*,*,#10555,.T.);
#14140=ORIENTED_EDGE('',*,*,#10698,.F.);
#14141=ORIENTED_EDGE('',*,*,#10545,.T.);
#14142=ORIENTED_EDGE('',*,*,#10651,.F.);
#14143=ORIENTED_EDGE('',*,*,#10551,.T.);
#14144=ORIENTED_EDGE('',*,*,#10699,.F.);
#14145=ORIENTED_EDGE('',*,*,#10541,.T.);
#14146=ORIENTED_EDGE('',*,*,#10652,.F.);
#14147=ORIENTED_EDGE('',*,*,#10547,.T.);
#14148=ORIENTED_EDGE('',*,*,#10700,.F.);
#14149=ORIENTED_EDGE('',*,*,#10537,.T.);
#14150=ORIENTED_EDGE('',*,*,#10653,.F.);
#14151=ORIENTED_EDGE('',*,*,#10543,.T.);
#14152=ORIENTED_EDGE('',*,*,#10701,.F.);
#14153=ORIENTED_EDGE('',*,*,#10533,.T.);
#14154=ORIENTED_EDGE('',*,*,#10654,.F.);
#14155=ORIENTED_EDGE('',*,*,#10539,.T.);
#14156=ORIENTED_EDGE('',*,*,#10702,.F.);
#14157=ORIENTED_EDGE('',*,*,#10529,.T.);
#14158=ORIENTED_EDGE('',*,*,#10655,.F.);
#14159=ORIENTED_EDGE('',*,*,#10535,.T.);
#14160=ORIENTED_EDGE('',*,*,#10703,.F.);
#14161=ORIENTED_EDGE('',*,*,#10525,.T.);
#14162=ORIENTED_EDGE('',*,*,#10656,.F.);
#14163=ORIENTED_EDGE('',*,*,#10531,.T.);
#14164=ORIENTED_EDGE('',*,*,#10704,.F.);
#14165=ORIENTED_EDGE('',*,*,#10521,.T.);
#14166=ORIENTED_EDGE('',*,*,#10657,.F.);
#14167=ORIENTED_EDGE('',*,*,#10527,.T.);
#14168=ORIENTED_EDGE('',*,*,#10705,.F.);
#14169=ORIENTED_EDGE('',*,*,#10517,.T.);
#14170=ORIENTED_EDGE('',*,*,#10658,.F.);
#14171=ORIENTED_EDGE('',*,*,#10523,.T.);
#14172=ORIENTED_EDGE('',*,*,#10706,.F.);
#14173=ORIENTED_EDGE('',*,*,#10513,.T.);
#14174=ORIENTED_EDGE('',*,*,#10659,.F.);
#14175=ORIENTED_EDGE('',*,*,#10519,.T.);
#14176=ORIENTED_EDGE('',*,*,#10707,.F.);
#14177=ORIENTED_EDGE('',*,*,#10509,.T.);
#14178=ORIENTED_EDGE('',*,*,#10660,.F.);
#14179=ORIENTED_EDGE('',*,*,#10515,.T.);
#14180=ORIENTED_EDGE('',*,*,#10708,.F.);
#14181=ORIENTED_EDGE('',*,*,#10505,.T.);
#14182=ORIENTED_EDGE('',*,*,#10661,.F.);
#14183=ORIENTED_EDGE('',*,*,#10511,.T.);
#14184=ORIENTED_EDGE('',*,*,#10709,.F.);
#14185=ORIENTED_EDGE('',*,*,#10501,.T.);
#14186=ORIENTED_EDGE('',*,*,#10662,.F.);
#14187=ORIENTED_EDGE('',*,*,#10507,.T.);
#14188=ORIENTED_EDGE('',*,*,#10710,.F.);
#14189=ORIENTED_EDGE('',*,*,#10497,.T.);
#14190=ORIENTED_EDGE('',*,*,#10663,.F.);
#14191=ORIENTED_EDGE('',*,*,#10503,.T.);
#14192=ORIENTED_EDGE('',*,*,#10711,.F.);
#14193=ORIENTED_EDGE('',*,*,#10493,.T.);
#14194=ORIENTED_EDGE('',*,*,#10664,.F.);
#14195=ORIENTED_EDGE('',*,*,#10499,.T.);
#14196=ORIENTED_EDGE('',*,*,#10712,.F.);
#14197=ORIENTED_EDGE('',*,*,#10489,.T.);
#14198=ORIENTED_EDGE('',*,*,#10665,.F.);
#14199=ORIENTED_EDGE('',*,*,#10495,.T.);
#14200=ORIENTED_EDGE('',*,*,#10713,.F.);
#14201=ORIENTED_EDGE('',*,*,#10485,.T.);
#14202=ORIENTED_EDGE('',*,*,#10666,.F.);
#14203=ORIENTED_EDGE('',*,*,#10491,.T.);
#14204=ORIENTED_EDGE('',*,*,#10714,.F.);
#14205=ORIENTED_EDGE('',*,*,#10481,.T.);
#14206=ORIENTED_EDGE('',*,*,#10667,.F.);
#14207=ORIENTED_EDGE('',*,*,#10487,.T.);
#14208=ORIENTED_EDGE('',*,*,#10715,.F.);
#14209=ORIENTED_EDGE('',*,*,#10477,.T.);
#14210=ORIENTED_EDGE('',*,*,#10668,.F.);
#14211=ORIENTED_EDGE('',*,*,#10483,.T.);
#14212=ORIENTED_EDGE('',*,*,#10716,.F.);
#14213=ORIENTED_EDGE('',*,*,#10473,.T.);
#14214=ORIENTED_EDGE('',*,*,#10669,.F.);
#14215=ORIENTED_EDGE('',*,*,#10479,.T.);
#14216=ORIENTED_EDGE('',*,*,#10717,.F.);
#14217=ORIENTED_EDGE('',*,*,#10469,.T.);
#14218=ORIENTED_EDGE('',*,*,#10670,.F.);
#14219=ORIENTED_EDGE('',*,*,#10475,.T.);
#14220=ORIENTED_EDGE('',*,*,#10718,.F.);
#14221=ORIENTED_EDGE('',*,*,#10465,.T.);
#14222=ORIENTED_EDGE('',*,*,#10671,.F.);
#14223=ORIENTED_EDGE('',*,*,#10471,.T.);
#14224=ORIENTED_EDGE('',*,*,#10719,.F.);
#14225=ORIENTED_EDGE('',*,*,#10461,.T.);
#14226=ORIENTED_EDGE('',*,*,#10672,.F.);
#14227=ORIENTED_EDGE('',*,*,#10467,.T.);
#14228=ORIENTED_EDGE('',*,*,#10720,.F.);
#14229=ORIENTED_EDGE('',*,*,#10457,.T.);
#14230=ORIENTED_EDGE('',*,*,#10673,.F.);
#14231=ORIENTED_EDGE('',*,*,#10463,.T.);
#14232=ORIENTED_EDGE('',*,*,#10721,.F.);
#14233=ORIENTED_EDGE('',*,*,#10677,.F.);
#14234=ORIENTED_EDGE('',*,*,#10722,.F.);
#14235=ORIENTED_EDGE('',*,*,#10678,.F.);
#14236=ORIENTED_EDGE('',*,*,#10630,.F.);
#14237=ORIENTED_EDGE('',*,*,#10454,.T.);
#14238=ORIENTED_EDGE('',*,*,#10723,.T.);
#14239=ORIENTED_EDGE('',*,*,#10458,.T.);
#14240=ORIENTED_EDGE('',*,*,#10721,.T.);
#14241=ORIENTED_EDGE('',*,*,#10462,.T.);
#14242=ORIENTED_EDGE('',*,*,#10720,.T.);
#14243=ORIENTED_EDGE('',*,*,#10466,.T.);
#14244=ORIENTED_EDGE('',*,*,#10719,.T.);
#14245=ORIENTED_EDGE('',*,*,#10470,.T.);
#14246=ORIENTED_EDGE('',*,*,#10718,.T.);
#14247=ORIENTED_EDGE('',*,*,#10474,.T.);
#14248=ORIENTED_EDGE('',*,*,#10717,.T.);
#14249=ORIENTED_EDGE('',*,*,#10478,.T.);
#14250=ORIENTED_EDGE('',*,*,#10716,.T.);
#14251=ORIENTED_EDGE('',*,*,#10482,.T.);
#14252=ORIENTED_EDGE('',*,*,#10715,.T.);
#14253=ORIENTED_EDGE('',*,*,#10486,.T.);
#14254=ORIENTED_EDGE('',*,*,#10714,.T.);
#14255=ORIENTED_EDGE('',*,*,#10490,.T.);
#14256=ORIENTED_EDGE('',*,*,#10713,.T.);
#14257=ORIENTED_EDGE('',*,*,#10494,.T.);
#14258=ORIENTED_EDGE('',*,*,#10712,.T.);
#14259=ORIENTED_EDGE('',*,*,#10498,.T.);
#14260=ORIENTED_EDGE('',*,*,#10711,.T.);
#14261=ORIENTED_EDGE('',*,*,#10502,.T.);
#14262=ORIENTED_EDGE('',*,*,#10710,.T.);
#14263=ORIENTED_EDGE('',*,*,#10506,.T.);
#14264=ORIENTED_EDGE('',*,*,#10709,.T.);
#14265=ORIENTED_EDGE('',*,*,#10510,.T.);
#14266=ORIENTED_EDGE('',*,*,#10708,.T.);
#14267=ORIENTED_EDGE('',*,*,#10514,.T.);
#14268=ORIENTED_EDGE('',*,*,#10707,.T.);
#14269=ORIENTED_EDGE('',*,*,#10518,.T.);
#14270=ORIENTED_EDGE('',*,*,#10706,.T.);
#14271=ORIENTED_EDGE('',*,*,#10522,.T.);
#14272=ORIENTED_EDGE('',*,*,#10705,.T.);
#14273=ORIENTED_EDGE('',*,*,#10526,.T.);
#14274=ORIENTED_EDGE('',*,*,#10704,.T.);
#14275=ORIENTED_EDGE('',*,*,#10530,.T.);
#14276=ORIENTED_EDGE('',*,*,#10703,.T.);
#14277=ORIENTED_EDGE('',*,*,#10534,.T.);
#14278=ORIENTED_EDGE('',*,*,#10702,.T.);
#14279=ORIENTED_EDGE('',*,*,#10538,.T.);
#14280=ORIENTED_EDGE('',*,*,#10701,.T.);
#14281=ORIENTED_EDGE('',*,*,#10542,.T.);
#14282=ORIENTED_EDGE('',*,*,#10700,.T.);
#14283=ORIENTED_EDGE('',*,*,#10546,.T.);
#14284=ORIENTED_EDGE('',*,*,#10699,.T.);
#14285=ORIENTED_EDGE('',*,*,#10550,.T.);
#14286=ORIENTED_EDGE('',*,*,#10698,.T.);
#14287=ORIENTED_EDGE('',*,*,#10554,.T.);
#14288=ORIENTED_EDGE('',*,*,#10697,.T.);
#14289=ORIENTED_EDGE('',*,*,#10558,.T.);
#14290=ORIENTED_EDGE('',*,*,#10696,.T.);
#14291=ORIENTED_EDGE('',*,*,#10562,.T.);
#14292=ORIENTED_EDGE('',*,*,#10695,.T.);
#14293=ORIENTED_EDGE('',*,*,#10566,.T.);
#14294=ORIENTED_EDGE('',*,*,#10694,.T.);
#14295=ORIENTED_EDGE('',*,*,#10570,.T.);
#14296=ORIENTED_EDGE('',*,*,#10693,.T.);
#14297=ORIENTED_EDGE('',*,*,#10574,.T.);
#14298=ORIENTED_EDGE('',*,*,#10692,.T.);
#14299=ORIENTED_EDGE('',*,*,#10578,.T.);
#14300=ORIENTED_EDGE('',*,*,#10691,.T.);
#14301=ORIENTED_EDGE('',*,*,#10582,.T.);
#14302=ORIENTED_EDGE('',*,*,#10690,.T.);
#14303=ORIENTED_EDGE('',*,*,#10586,.T.);
#14304=ORIENTED_EDGE('',*,*,#10689,.T.);
#14305=ORIENTED_EDGE('',*,*,#10590,.T.);
#14306=ORIENTED_EDGE('',*,*,#10688,.T.);
#14307=ORIENTED_EDGE('',*,*,#10594,.T.);
#14308=ORIENTED_EDGE('',*,*,#10687,.T.);
#14309=ORIENTED_EDGE('',*,*,#10598,.T.);
#14310=ORIENTED_EDGE('',*,*,#10686,.T.);
#14311=ORIENTED_EDGE('',*,*,#10602,.T.);
#14312=ORIENTED_EDGE('',*,*,#10685,.T.);
#14313=ORIENTED_EDGE('',*,*,#10606,.T.);
#14314=ORIENTED_EDGE('',*,*,#10684,.T.);
#14315=ORIENTED_EDGE('',*,*,#10610,.T.);
#14316=ORIENTED_EDGE('',*,*,#10683,.T.);
#14317=ORIENTED_EDGE('',*,*,#10614,.T.);
#14318=ORIENTED_EDGE('',*,*,#10682,.T.);
#14319=ORIENTED_EDGE('',*,*,#10618,.T.);
#14320=ORIENTED_EDGE('',*,*,#10681,.T.);
#14321=ORIENTED_EDGE('',*,*,#10622,.T.);
#14322=ORIENTED_EDGE('',*,*,#10680,.T.);
#14323=ORIENTED_EDGE('',*,*,#10626,.T.);
#14324=ORIENTED_EDGE('',*,*,#10679,.T.);
#14325=ORIENTED_EDGE('',*,*,#10722,.T.);
#14326=ORIENTED_EDGE('',*,*,#10676,.T.);
#14327=ORIENTED_EDGE('',*,*,#10724,.T.);
#14328=ORIENTED_EDGE('',*,*,#10453,.T.);
#14329=ORIENTED_EDGE('',*,*,#10674,.F.);
#14330=ORIENTED_EDGE('',*,*,#10459,.T.);
#14331=ORIENTED_EDGE('',*,*,#10723,.F.);
#14332=ORIENTED_EDGE('',*,*,#10724,.F.);
#14333=ORIENTED_EDGE('',*,*,#10725,.T.);
#14334=ORIENTED_EDGE('',*,*,#10675,.F.);
#14335=ORIENTED_EDGE('',*,*,#10725,.F.);
#18696=ADVANCED_FACE('',(#4980),#4339,.F.);
#18697=ADVANCED_FACE('',(#4981),#4340,.F.);
#18698=ADVANCED_FACE('',(#4982),#4341,.F.);
#18699=ADVANCED_FACE('',(#4983),#4342,.F.);
#18700=ADVANCED_FACE('',(#4984),#4343,.F.);
#18701=ADVANCED_FACE('',(#4985),#4344,.F.);
#18702=ADVANCED_FACE('',(#4986),#4345,.F.);
#18703=ADVANCED_FACE('',(#4987),#4346,.F.);
#18704=ADVANCED_FACE('',(#4988),#4347,.F.);
#18705=ADVANCED_FACE('',(#4989),#4348,.F.);
#18706=ADVANCED_FACE('',(#4990),#4349,.F.);
#18707=ADVANCED_FACE('',(#4991),#4350,.F.);
#18708=ADVANCED_FACE('',(#4992),#4351,.F.);
#18709=ADVANCED_FACE('',(#4993),#4352,.F.);
#18710=ADVANCED_FACE('',(#4994),#4353,.F.);
#18711=ADVANCED_FACE('',(#4995),#4354,.F.);
#18712=ADVANCED_FACE('',(#4996),#4355,.F.);
#18713=ADVANCED_FACE('',(#4997),#4356,.F.);
#18714=ADVANCED_FACE('',(#4998),#4357,.F.);
#18715=ADVANCED_FACE('',(#4999),#4358,.F.);
#18716=ADVANCED_FACE('',(#5000),#4359,.F.);
#18717=ADVANCED_FACE('',(#5001),#4360,.F.);
#18718=ADVANCED_FACE('',(#5002),#4361,.F.);
#18719=ADVANCED_FACE('',(#5003),#4362,.F.);
#18720=ADVANCED_FACE('',(#5004),#4363,.F.);
#18721=ADVANCED_FACE('',(#5005),#4364,.F.);
#18722=ADVANCED_FACE('',(#5006),#4365,.F.);
#18723=ADVANCED_FACE('',(#5007),#4366,.F.);
#18724=ADVANCED_FACE('',(#5008),#4367,.F.);
#18725=ADVANCED_FACE('',(#5009),#4368,.F.);
#18726=ADVANCED_FACE('',(#5010),#4369,.F.);
#18727=ADVANCED_FACE('',(#5011),#4370,.F.);
#18728=ADVANCED_FACE('',(#5012),#4371,.F.);
#18729=ADVANCED_FACE('',(#5013),#4372,.F.);
#18730=ADVANCED_FACE('',(#5014),#4373,.F.);
#18731=ADVANCED_FACE('',(#5015),#4374,.F.);
#18732=ADVANCED_FACE('',(#5016),#4375,.F.);
#18733=ADVANCED_FACE('',(#5017),#4376,.F.);
#18734=ADVANCED_FACE('',(#5018),#4377,.F.);
#18735=ADVANCED_FACE('',(#5019),#4378,.F.);
#18736=ADVANCED_FACE('',(#5020),#4379,.F.);
#18737=ADVANCED_FACE('',(#5021),#4380,.F.);
#18738=ADVANCED_FACE('',(#5022),#4381,.F.);
#18739=ADVANCED_FACE('',(#5023),#4382,.F.);
#18740=ADVANCED_FACE('',(#5024,#501),#717,.F.);
#18741=ADVANCED_FACE('',(#5025),#4383,.T.);
#18742=ADVANCED_FACE('',(#5026),#4384,.T.);
#18743=ADVANCED_FACE('',(#5027),#4385,.T.);
#18744=ADVANCED_FACE('',(#5028),#4386,.T.);
#18745=ADVANCED_FACE('',(#5029),#4387,.T.);
#18746=ADVANCED_FACE('',(#5030),#4388,.T.);
#18747=ADVANCED_FACE('',(#5031),#4389,.T.);
#18748=ADVANCED_FACE('',(#5032),#4390,.T.);
#18749=ADVANCED_FACE('',(#5033),#4391,.T.);
#18750=ADVANCED_FACE('',(#5034),#4392,.T.);
#18751=ADVANCED_FACE('',(#5035),#4393,.T.);
#18752=ADVANCED_FACE('',(#5036),#4394,.T.);
#18753=ADVANCED_FACE('',(#5037),#4395,.T.);
#18754=ADVANCED_FACE('',(#5038),#4396,.T.);
#18755=ADVANCED_FACE('',(#5039),#4397,.T.);
#18756=ADVANCED_FACE('',(#5040),#4398,.T.);
#18757=ADVANCED_FACE('',(#5041),#4399,.T.);
#18758=ADVANCED_FACE('',(#5042),#4400,.T.);
#18759=ADVANCED_FACE('',(#5043),#4401,.T.);
#18760=ADVANCED_FACE('',(#5044),#4402,.T.);
#18761=ADVANCED_FACE('',(#5045),#4403,.T.);
#18762=ADVANCED_FACE('',(#5046),#4404,.T.);
#18763=ADVANCED_FACE('',(#5047),#4405,.T.);
#18764=ADVANCED_FACE('',(#5048),#4406,.T.);
#18765=ADVANCED_FACE('',(#5049),#4407,.T.);
#18766=ADVANCED_FACE('',(#5050),#4408,.T.);
#18767=ADVANCED_FACE('',(#5051),#4409,.T.);
#18768=ADVANCED_FACE('',(#5052),#4410,.T.);
#18769=ADVANCED_FACE('',(#5053),#4411,.T.);
#18770=ADVANCED_FACE('',(#5054),#4412,.T.);
#18771=ADVANCED_FACE('',(#5055),#4413,.T.);
#18772=ADVANCED_FACE('',(#5056),#4414,.T.);
#18773=ADVANCED_FACE('',(#5057),#4415,.T.);
#18774=ADVANCED_FACE('',(#5058),#4416,.T.);
#18775=ADVANCED_FACE('',(#5059),#4417,.T.);
#18776=ADVANCED_FACE('',(#5060),#4418,.T.);
#18777=ADVANCED_FACE('',(#5061),#4419,.T.);
#18778=ADVANCED_FACE('',(#5062),#4420,.T.);
#18779=ADVANCED_FACE('',(#5063),#4421,.T.);
#18780=ADVANCED_FACE('',(#5064),#4422,.T.);
#18781=ADVANCED_FACE('',(#5065),#4423,.T.);
#18782=ADVANCED_FACE('',(#5066),#4424,.T.);
#18783=ADVANCED_FACE('',(#5067),#4425,.T.);
#18784=ADVANCED_FACE('',(#5068),#4426,.T.);
#18785=ADVANCED_FACE('',(#5069),#4427,.F.);
#18786=ADVANCED_FACE('',(#5070,#502),#718,.T.);
#18787=ADVANCED_FACE('',(#5071),#4428,.T.);
#18788=ADVANCED_FACE('',(#5072),#4429,.F.);
#19558=CLOSED_SHELL('',(#18696,#18697,#18698,#18699,#18700,#18701,#18702,
#18703,#18704,#18705,#18706,#18707,#18708,#18709,#18710,#18711,#18712,#18713,
#18714,#18715,#18716,#18717,#18718,#18719,#18720,#18721,#18722,#18723,#18724,
#18725,#18726,#18727,#18728,#18729,#18730,#18731,#18732,#18733,#18734,#18735,
#18736,#18737,#18738,#18739,#18740,#18741,#18742,#18743,#18744,#18745,#18746,
#18747,#18748,#18749,#18750,#18751,#18752,#18753,#18754,#18755,#18756,#18757,
#18758,#18759,#18760,#18761,#18762,#18763,#18764,#18765,#18766,#18767,#18768,
#18769,#18770,#18771,#18772,#18773,#18774,#18775,#18776,#18777,#18778,#18779,
#18780,#18781,#18782,#18783,#18784,#18785,#18786,#18787,#18788));
#20315=AXIS2_PLACEMENT_3D('',#29753,#23290,#23291);
#20316=AXIS2_PLACEMENT_3D('',#29754,#23292,#23293);
#20317=AXIS2_PLACEMENT_3D('',#29759,#23295,#23296);
#20318=AXIS2_PLACEMENT_3D('',#29762,#23298,#23299);
#20319=AXIS2_PLACEMENT_3D('',#29763,#23300,#23301);
#20320=AXIS2_PLACEMENT_3D('',#29768,#23303,#23304);
#20321=AXIS2_PLACEMENT_3D('',#29771,#23306,#23307);
#20322=AXIS2_PLACEMENT_3D('',#29772,#23308,#23309);
#20323=AXIS2_PLACEMENT_3D('',#29777,#23311,#23312);
#20324=AXIS2_PLACEMENT_3D('',#29780,#23314,#23315);
#20325=AXIS2_PLACEMENT_3D('',#29781,#23316,#23317);
#20326=AXIS2_PLACEMENT_3D('',#29786,#23319,#23320);
#20327=AXIS2_PLACEMENT_3D('',#29789,#23322,#23323);
#20328=AXIS2_PLACEMENT_3D('',#29790,#23324,#23325);
#20329=AXIS2_PLACEMENT_3D('',#29795,#23327,#23328);
#20330=AXIS2_PLACEMENT_3D('',#29798,#23330,#23331);
#20331=AXIS2_PLACEMENT_3D('',#29799,#23332,#23333);
#20332=AXIS2_PLACEMENT_3D('',#29804,#23335,#23336);
#20333=AXIS2_PLACEMENT_3D('',#29807,#23338,#23339);
#20334=AXIS2_PLACEMENT_3D('',#29808,#23340,#23341);
#20335=AXIS2_PLACEMENT_3D('',#29813,#23343,#23344);
#20336=AXIS2_PLACEMENT_3D('',#29816,#23346,#23347);
#20337=AXIS2_PLACEMENT_3D('',#29817,#23348,#23349);
#20338=AXIS2_PLACEMENT_3D('',#29822,#23351,#23352);
#20339=AXIS2_PLACEMENT_3D('',#29825,#23354,#23355);
#20340=AXIS2_PLACEMENT_3D('',#29826,#23356,#23357);
#20341=AXIS2_PLACEMENT_3D('',#29831,#23359,#23360);
#20342=AXIS2_PLACEMENT_3D('',#29834,#23362,#23363);
#20343=AXIS2_PLACEMENT_3D('',#29835,#23364,#23365);
#20344=AXIS2_PLACEMENT_3D('',#29840,#23367,#23368);
#20345=AXIS2_PLACEMENT_3D('',#29843,#23370,#23371);
#20346=AXIS2_PLACEMENT_3D('',#29844,#23372,#23373);
#20347=AXIS2_PLACEMENT_3D('',#29849,#23375,#23376);
#20348=AXIS2_PLACEMENT_3D('',#29852,#23378,#23379);
#20349=AXIS2_PLACEMENT_3D('',#29853,#23380,#23381);
#20350=AXIS2_PLACEMENT_3D('',#29858,#23383,#23384);
#20351=AXIS2_PLACEMENT_3D('',#29861,#23386,#23387);
#20352=AXIS2_PLACEMENT_3D('',#29862,#23388,#23389);
#20353=AXIS2_PLACEMENT_3D('',#29867,#23391,#23392);
#20354=AXIS2_PLACEMENT_3D('',#29870,#23394,#23395);
#20355=AXIS2_PLACEMENT_3D('',#29871,#23396,#23397);
#20356=AXIS2_PLACEMENT_3D('',#29876,#23399,#23400);
#20357=AXIS2_PLACEMENT_3D('',#29879,#23402,#23403);
#20358=AXIS2_PLACEMENT_3D('',#29880,#23404,#23405);
#20359=AXIS2_PLACEMENT_3D('',#29885,#23407,#23408);
#20360=AXIS2_PLACEMENT_3D('',#29888,#23410,#23411);
#20361=AXIS2_PLACEMENT_3D('',#29889,#23412,#23413);
#20362=AXIS2_PLACEMENT_3D('',#29894,#23415,#23416);
#20363=AXIS2_PLACEMENT_3D('',#29897,#23418,#23419);
#20364=AXIS2_PLACEMENT_3D('',#29898,#23420,#23421);
#20365=AXIS2_PLACEMENT_3D('',#29903,#23423,#23424);
#20366=AXIS2_PLACEMENT_3D('',#29906,#23426,#23427);
#20367=AXIS2_PLACEMENT_3D('',#29907,#23428,#23429);
#20368=AXIS2_PLACEMENT_3D('',#29912,#23431,#23432);
#20369=AXIS2_PLACEMENT_3D('',#29915,#23434,#23435);
#20370=AXIS2_PLACEMENT_3D('',#29916,#23436,#23437);
#20371=AXIS2_PLACEMENT_3D('',#29921,#23439,#23440);
#20372=AXIS2_PLACEMENT_3D('',#29924,#23442,#23443);
#20373=AXIS2_PLACEMENT_3D('',#29925,#23444,#23445);
#20374=AXIS2_PLACEMENT_3D('',#29930,#23447,#23448);
#20375=AXIS2_PLACEMENT_3D('',#29933,#23450,#23451);
#20376=AXIS2_PLACEMENT_3D('',#29934,#23452,#23453);
#20377=AXIS2_PLACEMENT_3D('',#29939,#23455,#23456);
#20378=AXIS2_PLACEMENT_3D('',#29942,#23458,#23459);
#20379=AXIS2_PLACEMENT_3D('',#29943,#23460,#23461);
#20380=AXIS2_PLACEMENT_3D('',#29948,#23463,#23464);
#20381=AXIS2_PLACEMENT_3D('',#29951,#23466,#23467);
#20382=AXIS2_PLACEMENT_3D('',#29952,#23468,#23469);
#20383=AXIS2_PLACEMENT_3D('',#29957,#23471,#23472);
#20384=AXIS2_PLACEMENT_3D('',#29960,#23474,#23475);
#20385=AXIS2_PLACEMENT_3D('',#29961,#23476,#23477);
#20386=AXIS2_PLACEMENT_3D('',#29966,#23479,#23480);
#20387=AXIS2_PLACEMENT_3D('',#29969,#23482,#23483);
#20388=AXIS2_PLACEMENT_3D('',#29970,#23484,#23485);
#20389=AXIS2_PLACEMENT_3D('',#29975,#23487,#23488);
#20390=AXIS2_PLACEMENT_3D('',#29978,#23490,#23491);
#20391=AXIS2_PLACEMENT_3D('',#29979,#23492,#23493);
#20392=AXIS2_PLACEMENT_3D('',#29984,#23495,#23496);
#20393=AXIS2_PLACEMENT_3D('',#29987,#23498,#23499);
#20394=AXIS2_PLACEMENT_3D('',#29988,#23500,#23501);
#20395=AXIS2_PLACEMENT_3D('',#29993,#23503,#23504);
#20396=AXIS2_PLACEMENT_3D('',#29996,#23506,#23507);
#20397=AXIS2_PLACEMENT_3D('',#29997,#23508,#23509);
#20398=AXIS2_PLACEMENT_3D('',#30002,#23511,#23512);
#20399=AXIS2_PLACEMENT_3D('',#30005,#23514,#23515);
#20400=AXIS2_PLACEMENT_3D('',#30006,#23516,#23517);
#20401=AXIS2_PLACEMENT_3D('',#30011,#23519,#23520);
#20402=AXIS2_PLACEMENT_3D('',#30014,#23522,#23523);
#20403=AXIS2_PLACEMENT_3D('',#30015,#23524,#23525);
#20404=AXIS2_PLACEMENT_3D('',#30020,#23527,#23528);
#20405=AXIS2_PLACEMENT_3D('',#30023,#23530,#23531);
#20406=AXIS2_PLACEMENT_3D('',#30024,#23532,#23533);
#20407=AXIS2_PLACEMENT_3D('',#30029,#23535,#23536);
#20408=AXIS2_PLACEMENT_3D('',#30032,#23538,#23539);
#20409=AXIS2_PLACEMENT_3D('',#30033,#23540,#23541);
#20410=AXIS2_PLACEMENT_3D('',#30038,#23543,#23544);
#20411=AXIS2_PLACEMENT_3D('',#30041,#23546,#23547);
#20412=AXIS2_PLACEMENT_3D('',#30042,#23548,#23549);
#20413=AXIS2_PLACEMENT_3D('',#30047,#23551,#23552);
#20414=AXIS2_PLACEMENT_3D('',#30050,#23554,#23555);
#20415=AXIS2_PLACEMENT_3D('',#30051,#23556,#23557);
#20416=AXIS2_PLACEMENT_3D('',#30056,#23559,#23560);
#20417=AXIS2_PLACEMENT_3D('',#30059,#23562,#23563);
#20418=AXIS2_PLACEMENT_3D('',#30060,#23564,#23565);
#20419=AXIS2_PLACEMENT_3D('',#30065,#23567,#23568);
#20420=AXIS2_PLACEMENT_3D('',#30068,#23570,#23571);
#20421=AXIS2_PLACEMENT_3D('',#30069,#23572,#23573);
#20422=AXIS2_PLACEMENT_3D('',#30074,#23575,#23576);
#20423=AXIS2_PLACEMENT_3D('',#30077,#23578,#23579);
#20424=AXIS2_PLACEMENT_3D('',#30078,#23580,#23581);
#20425=AXIS2_PLACEMENT_3D('',#30083,#23583,#23584);
#20426=AXIS2_PLACEMENT_3D('',#30086,#23586,#23587);
#20427=AXIS2_PLACEMENT_3D('',#30087,#23588,#23589);
#20428=AXIS2_PLACEMENT_3D('',#30092,#23591,#23592);
#20429=AXIS2_PLACEMENT_3D('',#30095,#23594,#23595);
#20430=AXIS2_PLACEMENT_3D('',#30096,#23596,#23597);
#20431=AXIS2_PLACEMENT_3D('',#30101,#23599,#23600);
#20432=AXIS2_PLACEMENT_3D('',#30104,#23602,#23603);
#20433=AXIS2_PLACEMENT_3D('',#30105,#23604,#23605);
#20434=AXIS2_PLACEMENT_3D('',#30110,#23607,#23608);
#20435=AXIS2_PLACEMENT_3D('',#30113,#23610,#23611);
#20436=AXIS2_PLACEMENT_3D('',#30114,#23612,#23613);
#20437=AXIS2_PLACEMENT_3D('',#30119,#23615,#23616);
#20438=AXIS2_PLACEMENT_3D('',#30122,#23618,#23619);
#20439=AXIS2_PLACEMENT_3D('',#30123,#23620,#23621);
#20440=AXIS2_PLACEMENT_3D('',#30128,#23623,#23624);
#20441=AXIS2_PLACEMENT_3D('',#30131,#23626,#23627);
#20442=AXIS2_PLACEMENT_3D('',#30132,#23628,#23629);
#20443=AXIS2_PLACEMENT_3D('',#30137,#23631,#23632);
#20444=AXIS2_PLACEMENT_3D('',#30140,#23634,#23635);
#20445=AXIS2_PLACEMENT_3D('',#30141,#23636,#23637);
#20446=AXIS2_PLACEMENT_3D('',#30146,#23639,#23640);
#20447=AXIS2_PLACEMENT_3D('',#30149,#23642,#23643);
#20448=AXIS2_PLACEMENT_3D('',#30150,#23644,#23645);
#20449=AXIS2_PLACEMENT_3D('',#30152,#23646,#23647);
#20450=AXIS2_PLACEMENT_3D('',#30154,#23648,#23649);
#20451=AXIS2_PLACEMENT_3D('',#30155,#23650,#23651);
#20452=AXIS2_PLACEMENT_3D('',#30156,#23652,#23653);
#20453=AXIS2_PLACEMENT_3D('',#30157,#23654,#23655);
#20454=AXIS2_PLACEMENT_3D('',#30158,#23656,#23657);
#20455=AXIS2_PLACEMENT_3D('',#30159,#23658,#23659);
#20456=AXIS2_PLACEMENT_3D('',#30160,#23660,#23661);
#20457=AXIS2_PLACEMENT_3D('',#30161,#23662,#23663);
#20458=AXIS2_PLACEMENT_3D('',#30162,#23664,#23665);
#20459=AXIS2_PLACEMENT_3D('',#30163,#23666,#23667);
#20460=AXIS2_PLACEMENT_3D('',#30164,#23668,#23669);
#20461=AXIS2_PLACEMENT_3D('',#30165,#23670,#23671);
#20462=AXIS2_PLACEMENT_3D('',#30166,#23672,#23673);
#20463=AXIS2_PLACEMENT_3D('',#30167,#23674,#23675);
#20464=AXIS2_PLACEMENT_3D('',#30168,#23676,#23677);
#20465=AXIS2_PLACEMENT_3D('',#30169,#23678,#23679);
#20466=AXIS2_PLACEMENT_3D('',#30170,#23680,#23681);
#20467=AXIS2_PLACEMENT_3D('',#30171,#23682,#23683);
#20468=AXIS2_PLACEMENT_3D('',#30172,#23684,#23685);
#20469=AXIS2_PLACEMENT_3D('',#30173,#23686,#23687);
#20470=AXIS2_PLACEMENT_3D('',#30174,#23688,#23689);
#20471=AXIS2_PLACEMENT_3D('',#30175,#23690,#23691);
#20472=AXIS2_PLACEMENT_3D('',#30176,#23692,#23693);
#20473=AXIS2_PLACEMENT_3D('',#30177,#23694,#23695);
#20474=AXIS2_PLACEMENT_3D('',#30178,#23696,#23697);
#20475=AXIS2_PLACEMENT_3D('',#30179,#23698,#23699);
#20476=AXIS2_PLACEMENT_3D('',#30180,#23700,#23701);
#20477=AXIS2_PLACEMENT_3D('',#30181,#23702,#23703);
#20478=AXIS2_PLACEMENT_3D('',#30182,#23704,#23705);
#20479=AXIS2_PLACEMENT_3D('',#30183,#23706,#23707);
#20480=AXIS2_PLACEMENT_3D('',#30184,#23708,#23709);
#20481=AXIS2_PLACEMENT_3D('',#30185,#23710,#23711);
#20482=AXIS2_PLACEMENT_3D('',#30186,#23712,#23713);
#20483=AXIS2_PLACEMENT_3D('',#30187,#23714,#23715);
#20484=AXIS2_PLACEMENT_3D('',#30188,#23716,#23717);
#20485=AXIS2_PLACEMENT_3D('',#30189,#23718,#23719);
#20486=AXIS2_PLACEMENT_3D('',#30190,#23720,#23721);
#20487=AXIS2_PLACEMENT_3D('',#30191,#23722,#23723);
#20488=AXIS2_PLACEMENT_3D('',#30192,#23724,#23725);
#20489=AXIS2_PLACEMENT_3D('',#30193,#23726,#23727);
#20490=AXIS2_PLACEMENT_3D('',#30194,#23728,#23729);
#20491=AXIS2_PLACEMENT_3D('',#30195,#23730,#23731);
#20492=AXIS2_PLACEMENT_3D('',#30196,#23732,#23733);
#20493=AXIS2_PLACEMENT_3D('',#30197,#23734,#23735);
#20494=AXIS2_PLACEMENT_3D('',#30198,#23736,#23737);
#20495=AXIS2_PLACEMENT_3D('',#30200,#23738,#23739);
#20496=AXIS2_PLACEMENT_3D('',#30201,#23740,#23741);
#20497=AXIS2_PLACEMENT_3D('',#30203,#23742,#23743);
#20498=AXIS2_PLACEMENT_3D('',#30205,#23745,#23746);
#20499=AXIS2_PLACEMENT_3D('',#30208,#23748,#23749);
#20500=AXIS2_PLACEMENT_3D('',#30209,#23750,#23751);
#20501=AXIS2_PLACEMENT_3D('',#30210,#23752,#23753);
#20502=AXIS2_PLACEMENT_3D('',#30211,#23754,#23755);
#20503=AXIS2_PLACEMENT_3D('',#30212,#23756,#23757);
#20504=AXIS2_PLACEMENT_3D('',#30213,#23758,#23759);
#20505=AXIS2_PLACEMENT_3D('',#30214,#23760,#23761);
#20506=AXIS2_PLACEMENT_3D('',#30215,#23762,#23763);
#20507=AXIS2_PLACEMENT_3D('',#30216,#23764,#23765);
#20508=AXIS2_PLACEMENT_3D('',#30217,#23766,#23767);
#20509=AXIS2_PLACEMENT_3D('',#30218,#23768,#23769);
#20510=AXIS2_PLACEMENT_3D('',#30219,#23770,#23771);
#20511=AXIS2_PLACEMENT_3D('',#30220,#23772,#23773);
#20512=AXIS2_PLACEMENT_3D('',#30221,#23774,#23775);
#20513=AXIS2_PLACEMENT_3D('',#30222,#23776,#23777);
#20514=AXIS2_PLACEMENT_3D('',#30223,#23778,#23779);
#20515=AXIS2_PLACEMENT_3D('',#30224,#23780,#23781);
#20516=AXIS2_PLACEMENT_3D('',#30225,#23782,#23783);
#20517=AXIS2_PLACEMENT_3D('',#30226,#23784,#23785);
#20518=AXIS2_PLACEMENT_3D('',#30227,#23786,#23787);
#20519=AXIS2_PLACEMENT_3D('',#30228,#23788,#23789);
#20520=AXIS2_PLACEMENT_3D('',#30229,#23790,#23791);
#20521=AXIS2_PLACEMENT_3D('',#30230,#23792,#23793);
#20522=AXIS2_PLACEMENT_3D('',#30231,#23794,#23795);
#20523=AXIS2_PLACEMENT_3D('',#30232,#23796,#23797);
#20524=AXIS2_PLACEMENT_3D('',#30233,#23798,#23799);
#20525=AXIS2_PLACEMENT_3D('',#30234,#23800,#23801);
#20526=AXIS2_PLACEMENT_3D('',#30235,#23802,#23803);
#20527=AXIS2_PLACEMENT_3D('',#30236,#23804,#23805);
#20528=AXIS2_PLACEMENT_3D('',#30237,#23806,#23807);
#20529=AXIS2_PLACEMENT_3D('',#30238,#23808,#23809);
#20530=AXIS2_PLACEMENT_3D('',#30239,#23810,#23811);
#20531=AXIS2_PLACEMENT_3D('',#30240,#23812,#23813);
#20532=AXIS2_PLACEMENT_3D('',#30241,#23814,#23815);
#20533=AXIS2_PLACEMENT_3D('',#30242,#23816,#23817);
#20534=AXIS2_PLACEMENT_3D('',#30243,#23818,#23819);
#20535=AXIS2_PLACEMENT_3D('',#30244,#23820,#23821);
#20536=AXIS2_PLACEMENT_3D('',#30245,#23822,#23823);
#20537=AXIS2_PLACEMENT_3D('',#30246,#23824,#23825);
#20538=AXIS2_PLACEMENT_3D('',#30247,#23826,#23827);
#20539=AXIS2_PLACEMENT_3D('',#30248,#23828,#23829);
#20540=AXIS2_PLACEMENT_3D('',#30249,#23830,#23831);
#20541=AXIS2_PLACEMENT_3D('',#30250,#23832,#23833);
#20542=AXIS2_PLACEMENT_3D('',#30251,#23834,#23835);
#20543=AXIS2_PLACEMENT_3D('',#30252,#23836,#23837);
#20544=AXIS2_PLACEMENT_3D('',#30253,#23838,#23839);
#20545=AXIS2_PLACEMENT_3D('',#30254,#23840,#23841);
#20546=AXIS2_PLACEMENT_3D('',#30255,#23842,#23843);
#20547=AXIS2_PLACEMENT_3D('',#30256,#23844,#23845);
#20548=AXIS2_PLACEMENT_3D('',#30257,#23846,#23847);
#20549=AXIS2_PLACEMENT_3D('',#30258,#23848,#23849);
#20550=AXIS2_PLACEMENT_3D('',#30259,#23850,#23851);
#20551=AXIS2_PLACEMENT_3D('',#30260,#23852,#23853);
#20552=AXIS2_PLACEMENT_3D('',#30261,#23854,#23855);
#20553=AXIS2_PLACEMENT_3D('',#30262,#23856,#23857);
#20554=AXIS2_PLACEMENT_3D('',#30263,#23858,#23859);
#20555=AXIS2_PLACEMENT_3D('',#30264,#23860,#23861);
#20556=AXIS2_PLACEMENT_3D('',#30265,#23862,#23863);
#20557=AXIS2_PLACEMENT_3D('',#30266,#23864,#23865);
#20558=AXIS2_PLACEMENT_3D('',#30267,#23866,#23867);
#20559=AXIS2_PLACEMENT_3D('',#30268,#23868,#23869);
#20560=AXIS2_PLACEMENT_3D('',#30269,#23870,#23871);
#20561=AXIS2_PLACEMENT_3D('',#30270,#23872,#23873);
#20562=AXIS2_PLACEMENT_3D('',#30271,#23874,#23875);
#20563=AXIS2_PLACEMENT_3D('',#30272,#23876,#23877);
#20564=AXIS2_PLACEMENT_3D('',#30273,#23878,#23879);
#20565=AXIS2_PLACEMENT_3D('',#30274,#23880,#23881);
#20566=AXIS2_PLACEMENT_3D('',#30275,#23882,#23883);
#20567=AXIS2_PLACEMENT_3D('',#30276,#23884,#23885);
#20568=AXIS2_PLACEMENT_3D('',#30277,#23886,#23887);
#20569=AXIS2_PLACEMENT_3D('',#30278,#23888,#23889);
#20570=AXIS2_PLACEMENT_3D('',#30279,#23890,#23891);
#20571=AXIS2_PLACEMENT_3D('',#30280,#23892,#23893);
#20572=AXIS2_PLACEMENT_3D('',#30281,#23894,#23895);
#20573=AXIS2_PLACEMENT_3D('',#30282,#23896,#23897);
#20574=AXIS2_PLACEMENT_3D('',#30283,#23898,#23899);
#20575=AXIS2_PLACEMENT_3D('',#30284,#23900,#23901);
#20576=AXIS2_PLACEMENT_3D('',#30285,#23902,#23903);
#20577=AXIS2_PLACEMENT_3D('',#30286,#23904,#23905);
#20578=AXIS2_PLACEMENT_3D('',#30287,#23906,#23907);
#20579=AXIS2_PLACEMENT_3D('',#30288,#23908,#23909);
#20580=AXIS2_PLACEMENT_3D('',#30289,#23910,#23911);
#20581=AXIS2_PLACEMENT_3D('',#30290,#23912,#23913);
#20582=AXIS2_PLACEMENT_3D('',#30291,#23914,#23915);
#20583=AXIS2_PLACEMENT_3D('',#30292,#23916,#23917);
#20584=AXIS2_PLACEMENT_3D('',#30293,#23918,#23919);
#20585=AXIS2_PLACEMENT_3D('',#30294,#23920,#23921);
#20586=AXIS2_PLACEMENT_3D('',#30295,#23922,#23923);
#20587=AXIS2_PLACEMENT_3D('',#30296,#23924,#23925);
#20588=AXIS2_PLACEMENT_3D('',#30298,#23926,#23927);
#20589=AXIS2_PLACEMENT_3D('',#30299,#23928,#23929);
#20590=AXIS2_PLACEMENT_3D('',#30300,#23930,#23931);
#23290=DIRECTION('axis',(0.,0.,1.));
#23291=DIRECTION('refdir',(1.,0.,0.));
#23292=DIRECTION('center_axis',(6.65798752924967E-17,-1.,1.71022579061586E-31));
#23293=DIRECTION('ref_axis',(-0.345824623417469,-2.30249603002096E-17,0.938299168622762));
#23294=DIRECTION('',(-6.65798752924967E-17,1.,-1.71022579061586E-31));
#23295=DIRECTION('center_axis',(-6.65798752924967E-17,1.,-1.71022579061586E-31));
#23296=DIRECTION('ref_axis',(-0.345824623433441,-2.3024960301273E-17,0.938299168616875));
#23297=DIRECTION('',(6.65798752924967E-17,-1.,1.71022579061586E-31));
#23298=DIRECTION('center_axis',(6.65798752924967E-17,-1.,1.71022579061586E-31));
#23299=DIRECTION('ref_axis',(-0.345824623433441,-2.3024960301273E-17,0.938299168616875));
#23300=DIRECTION('center_axis',(6.65798752924967E-17,-1.,1.71022579061586E-31));
#23301=DIRECTION('ref_axis',(-0.473045086880378,-3.14952828922237E-17,0.881038220384528));
#23302=DIRECTION('',(-6.65798752924967E-17,1.,-1.71022579061586E-31));
#23303=DIRECTION('center_axis',(-6.65798752924967E-17,1.,-1.71022579061586E-31));
#23304=DIRECTION('ref_axis',(-0.473045086892459,-3.1495282893028E-17,0.881038220378041));
#23305=DIRECTION('',(6.65798752924967E-17,-1.,1.71022579061586E-31));
#23306=DIRECTION('center_axis',(6.65798752924967E-17,-1.,1.71022579061586E-31));
#23307=DIRECTION('ref_axis',(-0.473045086892459,-3.1495282893028E-17,0.881038220378041));
#23308=DIRECTION('center_axis',(6.65798752924967E-17,-1.,1.71022579061586E-31));
#23309=DIRECTION('ref_axis',(-0.591058265807973,-3.93525856280941E-17,0.80662886535263));
#23310=DIRECTION('',(-6.65798752924967E-17,1.,-1.71022579061586E-31));
#23311=DIRECTION('center_axis',(-6.65798752924967E-17,1.,-1.71022579061586E-31));
#23312=DIRECTION('ref_axis',(-0.591058265816149,-3.93525856286384E-17,0.806628865346639));
#23313=DIRECTION('',(6.65798752924967E-17,-1.,1.71022579061586E-31));
#23314=DIRECTION('center_axis',(6.65798752924967E-17,-1.,1.71022579061586E-31));
#23315=DIRECTION('ref_axis',(-0.591058265816149,-3.93525856286384E-17,0.806628865346639));
#23316=DIRECTION('center_axis',(6.65798752924967E-17,-1.,1.71022579061586E-31));
#23317=DIRECTION('ref_axis',(-0.697567167910428,-4.64439350476163E-17,0.716519396983379));
#23318=DIRECTION('',(-6.65798752924967E-17,1.,-1.71022579061586E-31));
#23319=DIRECTION('center_axis',(-6.65798752924967E-17,1.,-1.71022579061586E-31));
#23320=DIRECTION('ref_axis',(-0.697567167914987,-4.64439350479198E-17,0.716519396978941));
#23321=DIRECTION('',(6.65798752924967E-17,-1.,1.71022579061586E-31));
#23322=DIRECTION('center_axis',(6.65798752924967E-17,-1.,1.71022579061586E-31));
#23323=DIRECTION('ref_axis',(-0.697567167914987,-4.64439350479198E-17,0.716519396978941));
#23324=DIRECTION('center_axis',(6.65798752924967E-17,-1.,1.71022579061586E-31));
#23325=DIRECTION('ref_axis',(-0.790498718560399,-5.26313061006297E-17,0.61246369358058));
#23326=DIRECTION('',(-6.65798752924967E-17,1.,-1.71022579061586E-31));
#23327=DIRECTION('center_axis',(-6.65798752924967E-17,1.,-1.71022579061586E-31));
#23328=DIRECTION('ref_axis',(-0.790498718561909,-5.26313061007302E-17,0.612463693578632));
#23329=DIRECTION('',(6.65798752924967E-17,-1.,1.71022579061586E-31));
#23330=DIRECTION('center_axis',(6.65798752924967E-17,-1.,1.71022579061586E-31));
#23331=DIRECTION('ref_axis',(-0.790498718561909,-5.26313061007302E-17,0.612463693578632));
#23332=DIRECTION('center_axis',(6.65798752924967E-17,-1.,1.71022579061586E-31));
#23333=DIRECTION('ref_axis',(-0.868044110832557,-5.77942686476178E-17,0.496487081049362));
#23334=DIRECTION('',(-6.65798752924967E-17,1.,-1.71022579061586E-31));
#23335=DIRECTION('center_axis',(-6.65798752924967E-17,1.,-1.71022579061586E-31));
#23336=DIRECTION('ref_axis',(-0.868044110831822,-5.77942686475688E-17,0.496487081050647));
#23337=DIRECTION('',(6.65798752924967E-17,-1.,1.71022579061586E-31));
#23338=DIRECTION('center_axis',(6.65798752924967E-17,-1.,1.71022579061586E-31));
#23339=DIRECTION('ref_axis',(-0.868044110831822,-5.77942686475688E-17,0.496487081050647));
#23340=DIRECTION('center_axis',(6.65798752924967E-17,-1.,1.71022579061586E-31));
#23341=DIRECTION('ref_axis',(-0.928694011872901,-6.18323314953861E-17,0.370846912231201));
#23342=DIRECTION('',(-6.65798752924967E-17,1.,-1.71022579061586E-31));
#23343=DIRECTION('center_axis',(-6.65798752924967E-17,1.,-1.71022579061586E-31));
#23344=DIRECTION('ref_axis',(-0.9286940118709,-6.18323314952529E-17,0.370846912236213));
#23345=DIRECTION('',(6.65798752924967E-17,-1.,1.71022579061586E-31));
#23346=DIRECTION('center_axis',(6.65798752924967E-17,-1.,1.71022579061586E-31));
#23347=DIRECTION('ref_axis',(-0.9286940118709,-6.18323314952529E-17,0.370846912236213));
#23348=DIRECTION('center_axis',(6.65798752924967E-17,-1.,1.71022579061586E-31));
#23349=DIRECTION('ref_axis',(-0.97126794034592,-6.46668983438314E-17,0.237988630098571));
#23350=DIRECTION('',(-6.65798752924967E-17,1.,-1.71022579061586E-31));
#23351=DIRECTION('center_axis',(-6.65798752924967E-17,1.,-1.71022579061586E-31));
#23352=DIRECTION('ref_axis',(-0.971267940343728,-6.46668983436855E-17,0.237988630107515));
#23353=DIRECTION('',(6.65798752924967E-17,-1.,1.71022579061586E-31));
#23354=DIRECTION('center_axis',(6.65798752924967E-17,-1.,1.71022579061586E-31));
#23355=DIRECTION('ref_axis',(-0.971267940343728,-6.46668983436855E-17,0.237988630107515));
#23356=DIRECTION('center_axis',(6.65798752924967E-17,-1.,1.71022579061586E-31));
#23357=DIRECTION('ref_axis',(-0.994937243161013,-6.62427975735207E-17,0.100498169989126));
#23358=DIRECTION('',(-6.65798752924967E-17,1.,-1.71022579061586E-31));
#23359=DIRECTION('center_axis',(-6.65798752924967E-17,1.,-1.71022579061586E-31));
#23360=DIRECTION('ref_axis',(-0.994937243159722,-6.62427975734348E-17,0.100498170001902));
#23361=DIRECTION('',(6.65798752924967E-17,-1.,1.71022579061586E-31));
#23362=DIRECTION('center_axis',(6.65798752924967E-17,-1.,1.71022579061586E-31));
#23363=DIRECTION('ref_axis',(-0.994937243159722,-6.62427975734348E-17,0.100498170001902));
#23364=DIRECTION('center_axis',(6.65798752924967E-17,-1.,1.71022579061586E-31));
#23365=DIRECTION('ref_axis',(-0.999241224262317,-6.65293560985068E-17,-0.0389483726841831));
#23366=DIRECTION('',(-6.65798752924967E-17,1.,-1.71022579061586E-31));
#23367=DIRECTION('center_axis',(-6.65798752924967E-17,1.,-1.71022579061586E-31));
#23368=DIRECTION('ref_axis',(-0.999241224262949,-6.65293560985489E-17,-0.038948372667972));
#23369=DIRECTION('',(6.65798752924967E-17,-1.,1.71022579061586E-31));
#23370=DIRECTION('center_axis',(6.65798752924967E-17,-1.,1.71022579061586E-31));
#23371=DIRECTION('ref_axis',(-0.999241224262949,-6.65293560985489E-17,-0.038948372667972));
#23372=DIRECTION('center_axis',(6.65798752924967E-17,-1.,1.71022579061586E-31));
#23373=DIRECTION('ref_axis',(-0.984096111553401,-6.55209963830564E-17,-0.177636829586311));
#23374=DIRECTION('',(-6.65798752924967E-17,1.,-1.71022579061586E-31));
#23375=DIRECTION('center_axis',(-6.65798752924967E-17,1.,-1.71022579061586E-31));
#23376=DIRECTION('ref_axis',(-0.984096111556828,-6.55209963832845E-17,-0.177636829567328));
#23377=DIRECTION('',(6.65798752924967E-17,-1.,1.71022579061586E-31));
#23378=DIRECTION('center_axis',(6.65798752924967E-17,-1.,1.71022579061586E-31));
#23379=DIRECTION('ref_axis',(-0.984096111556828,-6.55209963832845E-17,-0.177636829567328));
#23380=DIRECTION('center_axis',(6.65798752924967E-17,-1.,1.71022579061586E-31));
#23381=DIRECTION('ref_axis',(-0.949796687425834,-6.32373450020385E-17,-0.312867787659441));
#23382=DIRECTION('',(-6.65798752924967E-17,1.,-1.71022579061586E-31));
#23383=DIRECTION('center_axis',(-6.65798752924967E-17,1.,-1.71022579061586E-31));
#23384=DIRECTION('ref_axis',(-0.949796687420265,-6.32373450016678E-17,-0.312867787676347));
#23385=DIRECTION('',(6.65798752924967E-17,-1.,1.71022579061586E-31));
#23386=DIRECTION('center_axis',(6.65798752924967E-17,-1.,1.71022579061586E-31));
#23387=DIRECTION('ref_axis',(-0.949796687420265,-6.32373450016678E-17,-0.312867787676347));
#23388=DIRECTION('center_axis',(6.65798752924967E-17,-1.,1.71022579061586E-31));
#23389=DIRECTION('ref_axis',(-0.897010551155241,-5.97228506319698E-17,-0.442009130127614));
#23390=DIRECTION('',(-6.65798752924967E-17,1.,-1.71022579061586E-31));
#23391=DIRECTION('center_axis',(-6.65798752924967E-17,1.,-1.71022579061586E-31));
#23392=DIRECTION('ref_axis',(-0.897010551148803,-5.97228506315411E-17,-0.442009130140681));
#23393=DIRECTION('',(6.65798752924967E-17,-1.,1.71022579061586E-31));
#23394=DIRECTION('center_axis',(6.65798752924967E-17,-1.,1.71022579061586E-31));
#23395=DIRECTION('ref_axis',(-0.897010551148803,-5.97228506315411E-17,-0.442009130140681));
#23396=DIRECTION('center_axis',(6.65798752924967E-17,-1.,1.71022579061586E-31));
#23397=DIRECTION('ref_axis',(-0.826765124840791,-5.50459189080855E-17,-0.562547267655786));
#23398=DIRECTION('',(-6.65798752924967E-17,1.,-1.71022579061586E-31));
#23399=DIRECTION('center_axis',(-6.65798752924967E-17,1.,-1.71022579061586E-31));
#23400=DIRECTION('ref_axis',(-0.826765124834574,-5.50459189076715E-17,-0.562547267664923));
#23401=DIRECTION('',(6.65798752924967E-17,-1.,1.71022579061586E-31));
#23402=DIRECTION('center_axis',(6.65798752924967E-17,-1.,1.71022579061586E-31));
#23403=DIRECTION('ref_axis',(-0.826765124834574,-5.50459189076715E-17,-0.562547267664923));
#23404=DIRECTION('center_axis',(6.65798752924967E-17,-1.,1.71022579061586E-31));
#23405=DIRECTION('ref_axis',(-0.740427655802706,-4.929758098646E-17,-0.672136062507071));
#23406=DIRECTION('',(-6.65798752924967E-17,1.,-1.71022579061586E-31));
#23407=DIRECTION('center_axis',(-6.65798752924967E-17,1.,-1.71022579061586E-31));
#23408=DIRECTION('ref_axis',(-0.740427655797785,-4.92975809861323E-17,-0.672136062512493));
#23409=DIRECTION('',(6.65798752924967E-17,-1.,1.71022579061586E-31));
#23410=DIRECTION('center_axis',(6.65798752924967E-17,-1.,1.71022579061586E-31));
#23411=DIRECTION('ref_axis',(-0.740427655797785,-4.92975809861323E-17,-0.672136062512493));
#23412=DIRECTION('center_axis',(6.65798752924967E-17,-1.,1.71022579061586E-31));
#23413=DIRECTION('ref_axis',(-0.639678604668397,-4.25897217261003E-17,-0.768642493445095));
#23414=DIRECTION('',(-6.65798752924967E-17,1.,-1.71022579061586E-31));
#23415=DIRECTION('center_axis',(-6.65798752924967E-17,1.,-1.71022579061586E-31));
#23416=DIRECTION('ref_axis',(-0.639678604665747,-4.25897217259239E-17,-0.7686424934473));
#23417=DIRECTION('',(6.65798752924967E-17,-1.,1.71022579061586E-31));
#23418=DIRECTION('center_axis',(6.65798752924967E-17,-1.,1.71022579061586E-31));
#23419=DIRECTION('ref_axis',(-0.639678604665747,-4.25897217259239E-17,-0.7686424934473));
#23420=DIRECTION('center_axis',(6.65798752924967E-17,-1.,1.71022579061586E-31));
#23421=DIRECTION('ref_axis',(-0.526478937117844,-3.50529019774324E-17,-0.850188172566088));
#23422=DIRECTION('',(-6.65798752924967E-17,1.,-1.71022579061586E-31));
#23423=DIRECTION('center_axis',(-6.65798752924967E-17,1.,-1.71022579061586E-31));
#23424=DIRECTION('ref_axis',(-0.526478937118264,-3.50529019774604E-17,-0.850188172565828));
#23425=DIRECTION('',(6.65798752924967E-17,-1.,1.71022579061586E-31));
#23426=DIRECTION('center_axis',(6.65798752924967E-17,-1.,1.71022579061586E-31));
#23427=DIRECTION('ref_axis',(-0.526478937118264,-3.50529019774604E-17,-0.850188172565828));
#23428=DIRECTION('center_axis',(6.65798752924967E-17,-1.,1.71022579061586E-31));
#23429=DIRECTION('ref_axis',(-0.403031955917209,-2.6833817363859E-17,-0.915185905982795));
#23430=DIRECTION('',(-6.65798752924967E-17,1.,-1.71022579061586E-31));
#23431=DIRECTION('center_axis',(-6.65798752924967E-17,1.,-1.71022579061586E-31));
#23432=DIRECTION('ref_axis',(-0.403031955921259,-2.68338173641286E-17,-0.915185905981011));
#23433=DIRECTION('',(6.65798752924967E-17,-1.,1.71022579061586E-31));
#23434=DIRECTION('center_axis',(6.65798752924967E-17,-1.,1.71022579061586E-31));
#23435=DIRECTION('ref_axis',(-0.403031955921259,-2.68338173641286E-17,-0.915185905981011));
#23436=DIRECTION('center_axis',(6.65798752924967E-17,-1.,1.71022579061586E-31));
#23437=DIRECTION('ref_axis',(-0.2717404161367,-1.80924430183128E-17,-0.962370586748085));
#23438=DIRECTION('',(-6.65798752924967E-17,1.,-1.71022579061586E-31));
#23439=DIRECTION('center_axis',(-6.65798752924967E-17,1.,-1.71022579061586E-31));
#23440=DIRECTION('ref_axis',(-0.271740416144659,-1.80924430188427E-17,-0.962370586745838));
#23441=DIRECTION('',(6.65798752924967E-17,-1.,1.71022579061586E-31));
#23442=DIRECTION('center_axis',(6.65798752924967E-17,-1.,1.71022579061586E-31));
#23443=DIRECTION('ref_axis',(-0.271740416144659,-1.80924430188427E-17,-0.962370586745838));
#23444=DIRECTION('center_axis',(6.65798752924967E-17,-1.,1.71022579061586E-31));
#23445=DIRECTION('ref_axis',(-0.135159758256232,-8.9989198492641E-18,-0.990823818722641));
#23446=DIRECTION('',(-6.65798752924967E-17,1.,-1.71022579061586E-31));
#23447=DIRECTION('center_axis',(-6.65798752924967E-17,1.,-1.71022579061586E-31));
#23448=DIRECTION('ref_axis',(-0.135159758268076,-8.99891985005266E-18,-0.990823818721025));
#23449=DIRECTION('',(6.65798752924967E-17,-1.,1.71022579061586E-31));
#23450=DIRECTION('center_axis',(6.65798752924967E-17,-1.,1.71022579061586E-31));
#23451=DIRECTION('ref_axis',(-0.135159758268076,-8.99891985005266E-18,-0.990823818721025));
#23452=DIRECTION('center_axis',(6.65798752924967E-17,-1.,1.71022579061586E-31));
#23453=DIRECTION('ref_axis',(0.00405163057674682,2.69757058530899E-19,-0.99999179211115));
#23454=DIRECTION('',(-6.65798752924967E-17,1.,-1.71022579061586E-31));
#23455=DIRECTION('center_axis',(-6.65798752924967E-17,1.,-1.71022579061586E-31));
#23456=DIRECTION('ref_axis',(0.00405163056134247,2.69757057505279E-19,-0.999991792111212));
#23457=DIRECTION('',(6.65798752924967E-17,-1.,1.71022579061586E-31));
#23458=DIRECTION('center_axis',(6.65798752924967E-17,-1.,1.71022579061586E-31));
#23459=DIRECTION('ref_axis',(0.00405163056134247,2.69757057505279E-19,-0.999991792111212));
#23460=DIRECTION('center_axis',(6.65798752924967E-17,-1.,1.71022579061586E-31));
#23461=DIRECTION('ref_axis',(0.143184159029212,9.53318345202578E-18,-0.98969606274002));
#23462=DIRECTION('',(-6.65798752924967E-17,1.,-1.71022579061586E-31));
#23463=DIRECTION('center_axis',(-6.65798752924967E-17,1.,-1.71022579061586E-31));
#23464=DIRECTION('ref_axis',(0.143184159010847,9.53318345080304E-18,-0.989696062742677));
#23465=DIRECTION('',(6.65798752924967E-17,-1.,1.71022579061586E-31));
#23466=DIRECTION('center_axis',(6.65798752924967E-17,-1.,1.71022579061586E-31));
#23467=DIRECTION('ref_axis',(0.143184159010847,9.53318345080304E-18,-0.989696062742677));
#23468=DIRECTION('center_axis',(6.65798752924967E-17,-1.,1.71022579061586E-31));
#23469=DIRECTION('ref_axis',(0.27952977069574,1.86110572734624E-17,-0.960137025270241));
#23470=DIRECTION('',(-6.65798752924967E-17,1.,-1.71022579061586E-31));
#23471=DIRECTION('center_axis',(-6.65798752924967E-17,1.,-1.71022579061586E-31));
#23472=DIRECTION('ref_axis',(0.279529770713557,1.86110572746487E-17,-0.960137025265054));
#23473=DIRECTION('',(6.65798752924967E-17,-1.,1.71022579061586E-31));
#23474=DIRECTION('center_axis',(6.65798752924967E-17,-1.,1.71022579061586E-31));
#23475=DIRECTION('ref_axis',(0.279529770713557,1.86110572746487E-17,-0.960137025265054));
#23476=DIRECTION('center_axis',(6.65798752924967E-17,-1.,1.71022579061586E-31));
#23477=DIRECTION('ref_axis',(0.410434653336076,2.73266880348349E-17,-0.911890012743256));
#23478=DIRECTION('',(-6.65798752924967E-17,1.,-1.71022579061586E-31));
#23479=DIRECTION('center_axis',(-6.65798752924967E-17,1.,-1.71022579061586E-31));
#23480=DIRECTION('ref_axis',(0.410434653350123,2.73266880357702E-17,-0.911890012736933));
#23481=DIRECTION('',(6.65798752924967E-17,-1.,1.71022579061586E-31));
#23482=DIRECTION('center_axis',(6.65798752924967E-17,-1.,1.71022579061586E-31));
#23483=DIRECTION('ref_axis',(0.410434653350123,2.73266880357702E-17,-0.911890012736933));
#23484=DIRECTION('center_axis',(6.65798752924967E-17,-1.,1.71022579061586E-31));
#23485=DIRECTION('ref_axis',(0.533350892311725,3.55104358972563E-17,-0.845894098377738));
#23486=DIRECTION('',(-6.65798752924967E-17,1.,-1.71022579061586E-31));
#23487=DIRECTION('center_axis',(-6.65798752924967E-17,1.,-1.71022579061586E-31));
#23488=DIRECTION('ref_axis',(0.533350892321836,3.55104358979295E-17,-0.845894098371363));
#23489=DIRECTION('',(6.65798752924967E-17,-1.,1.71022579061586E-31));
#23490=DIRECTION('center_axis',(6.65798752924967E-17,-1.,1.71022579061586E-31));
#23491=DIRECTION('ref_axis',(0.533350892321836,3.55104358979295E-17,-0.845894098371363));
#23492=DIRECTION('center_axis',(6.65798752924967E-17,-1.,1.71022579061586E-31));
#23493=DIRECTION('ref_axis',(0.645886062846174,4.30030135174598E-17,-0.763433817577574));
#23494=DIRECTION('',(-6.65798752924967E-17,1.,-1.71022579061586E-31));
#23495=DIRECTION('center_axis',(-6.65798752924967E-17,1.,-1.71022579061586E-31));
#23496=DIRECTION('ref_axis',(0.645886062852486,4.30030135178801E-17,-0.763433817572233));
#23497=DIRECTION('',(6.65798752924967E-17,-1.,1.71022579061586E-31));
#23498=DIRECTION('center_axis',(6.65798752924967E-17,-1.,1.71022579061586E-31));
#23499=DIRECTION('ref_axis',(0.645886062852486,4.30030135178801E-17,-0.763433817572233));
#23500=DIRECTION('center_axis',(6.65798752924967E-17,-1.,1.71022579061586E-31));
#23501=DIRECTION('ref_axis',(0.745849795851828,4.96585863947487E-17,-0.666114165911359));
#23502=DIRECTION('',(-6.65798752924967E-17,1.,-1.71022579061586E-31));
#23503=DIRECTION('center_axis',(-6.65798752924967E-17,1.,-1.71022579061586E-31));
#23504=DIRECTION('ref_axis',(0.745849795854776,4.9658586394945E-17,-0.66611416590806));
#23505=DIRECTION('',(6.65798752924967E-17,-1.,1.71022579061586E-31));
#23506=DIRECTION('center_axis',(6.65798752924967E-17,-1.,1.71022579061586E-31));
#23507=DIRECTION('ref_axis',(0.745849795854776,4.9658586394945E-17,-0.66611416590806));
#23508=DIRECTION('center_axis',(6.65798752924967E-17,-1.,1.71022579061586E-31));
#23509=DIRECTION('ref_axis',(0.831296410972796,5.53476113736688E-17,-0.555829359699313));
#23510=DIRECTION('',(-6.65798752924967E-17,1.,-1.71022579061586E-31));
#23511=DIRECTION('center_axis',(-6.65798752924967E-17,1.,-1.71022579061586E-31));
#23512=DIRECTION('ref_axis',(0.83129641097307,5.5347611373687E-17,-0.555829359698903));
#23513=DIRECTION('',(6.65798752924967E-17,-1.,1.71022579061586E-31));
#23514=DIRECTION('center_axis',(6.65798752924967E-17,-1.,1.71022579061586E-31));
#23515=DIRECTION('ref_axis',(0.83129641097307,5.5347611373687E-17,-0.555829359698903));
#23516=DIRECTION('center_axis',(6.65798752924967E-17,-1.,1.71022579061586E-31));
#23517=DIRECTION('ref_axis',(0.900562787039831,5.99593580541751E-17,-0.434725967247245));
#23518=DIRECTION('',(-6.65798752924967E-17,1.,-1.71022579061586E-31));
#23519=DIRECTION('center_axis',(-6.65798752924967E-17,1.,-1.71022579061586E-31));
#23520=DIRECTION('ref_axis',(0.900562787038332,5.99593580540753E-17,-0.434725967250349));
#23521=DIRECTION('',(6.65798752924967E-17,-1.,1.71022579061586E-31));
#23522=DIRECTION('center_axis',(6.65798752924967E-17,-1.,1.71022579061586E-31));
#23523=DIRECTION('ref_axis',(0.900562787038332,5.99593580540753E-17,-0.434725967250349));
#23524=DIRECTION('center_axis',(6.65798752924967E-17,-1.,1.71022579061586E-31));
#23525=DIRECTION('ref_axis',(0.952300732832122,6.34040640329159E-17,-0.305161128336168));
#23526=DIRECTION('',(-6.65798752924967E-17,1.,-1.71022579061586E-31));
#23527=DIRECTION('center_axis',(-6.65798752924967E-17,1.,-1.71022579061586E-31));
#23528=DIRECTION('ref_axis',(0.952300732829888,6.34040640327671E-17,-0.30516112834314));
#23529=DIRECTION('',(6.65798752924967E-17,-1.,1.71022579061586E-31));
#23530=DIRECTION('center_axis',(6.65798752924967E-17,-1.,1.71022579061586E-31));
#23531=DIRECTION('ref_axis',(0.952300732829888,6.34040640327671E-17,-0.30516112834314));
#23532=DIRECTION('center_axis',(6.65798752924967E-17,-1.,1.71022579061586E-31));
#23533=DIRECTION('ref_axis',(0.985503228085865,6.56146820263098E-17,-0.169656675177667));
#23534=DIRECTION('',(-6.65798752924967E-17,1.,-1.71022579061586E-31));
#23535=DIRECTION('center_axis',(-6.65798752924967E-17,1.,-1.71022579061586E-31));
#23536=DIRECTION('ref_axis',(0.985503228083989,6.56146820261849E-17,-0.169656675188558));
#23537=DIRECTION('',(6.65798752924967E-17,-1.,1.71022579061586E-31));
#23538=DIRECTION('center_axis',(6.65798752924967E-17,-1.,1.71022579061586E-31));
#23539=DIRECTION('ref_axis',(0.985503228083989,6.56146820261849E-17,-0.169656675188558));
#23540=DIRECTION('center_axis',(6.65798752924967E-17,-1.,1.71022579061586E-31));
#23541=DIRECTION('ref_axis',(0.999524023998223,6.65481848696562E-17,-0.0308500478184399));
#23542=DIRECTION('',(-6.65798752924967E-17,1.,-1.71022579061586E-31));
#23543=DIRECTION('center_axis',(-6.65798752924967E-17,1.,-1.71022579061586E-31));
#23544=DIRECTION('ref_axis',(0.999524023997774,6.65481848696262E-17,-0.0308500478330001));
#23545=DIRECTION('',(6.65798752924967E-17,-1.,1.71022579061586E-31));
#23546=DIRECTION('center_axis',(6.65798752924967E-17,-1.,1.71022579061586E-31));
#23547=DIRECTION('ref_axis',(0.999524023997774,6.65481848696262E-17,-0.0308500478330001));
#23548=DIRECTION('center_axis',(6.65798752924967E-17,-1.,1.71022579061586E-31));
#23549=DIRECTION('ref_axis',(0.994090221725182,6.6186402991953E-17,0.108557040630164));
#23550=DIRECTION('',(-6.65798752924967E-17,1.,-1.71022579061586E-31));
#23551=DIRECTION('center_axis',(-6.65798752924967E-17,1.,-1.71022579061586E-31));
#23552=DIRECTION('ref_axis',(0.994090221727114,6.61864029920817E-17,0.108557040612469));
#23553=DIRECTION('',(6.65798752924967E-17,-1.,1.71022579061586E-31));
#23554=DIRECTION('center_axis',(6.65798752924967E-17,-1.,1.71022579061586E-31));
#23555=DIRECTION('ref_axis',(0.994090221727114,6.61864029920817E-17,0.108557040612469));
#23556=DIRECTION('center_axis',(6.65798752924967E-17,-1.,1.71022579061586E-31));
#23557=DIRECTION('ref_axis',(0.969307584047127,6.4536378065929E-17,0.245851189764706));
#23558=DIRECTION('',(-6.65798752924967E-17,1.,-1.71022579061586E-31));
#23559=DIRECTION('center_axis',(-6.65798752924967E-17,1.,-1.71022579061586E-31));
#23560=DIRECTION('ref_axis',(0.969307584042385,6.45363780656133E-17,0.245851189783404));
#23561=DIRECTION('',(6.65798752924967E-17,-1.,1.71022579061586E-31));
#23562=DIRECTION('center_axis',(6.65798752924967E-17,-1.,1.71022579061586E-31));
#23563=DIRECTION('ref_axis',(0.969307584042385,6.45363780656133E-17,0.245851189783404));
#23564=DIRECTION('center_axis',(6.65798752924967E-17,-1.,1.71022579061586E-31));
#23565=DIRECTION('ref_axis',(0.925658476816631,6.16302259498938E-17,0.37836012514206));
#23566=DIRECTION('',(-6.65798752924967E-17,1.,-1.71022579061586E-31));
#23567=DIRECTION('center_axis',(-6.65798752924967E-17,1.,-1.71022579061586E-31));
#23568=DIRECTION('ref_axis',(0.925658476810492,6.16302259494851E-17,0.378360125157078));
#23569=DIRECTION('',(6.65798752924967E-17,-1.,1.71022579061586E-31));
#23570=DIRECTION('center_axis',(6.65798752924967E-17,-1.,1.71022579061586E-31));
#23571=DIRECTION('ref_axis',(0.925658476810492,6.16302259494851E-17,0.378360125157078));
#23572=DIRECTION('center_axis',(6.65798752924967E-17,-1.,1.71022579061586E-31));
#23573=DIRECTION('ref_axis',(0.86399248025581,5.75245115890868E-17,0.503504711061788));
#23574=DIRECTION('',(-6.65798752924967E-17,1.,-1.71022579061586E-31));
#23575=DIRECTION('center_axis',(-6.65798752924967E-17,1.,-1.71022579061586E-31));
#23576=DIRECTION('ref_axis',(0.863992480249344,5.75245115886563E-17,0.503504711072882));
#23577=DIRECTION('',(6.65798752924967E-17,-1.,1.71022579061586E-31));
#23578=DIRECTION('center_axis',(6.65798752924967E-17,-1.,1.71022579061586E-31));
#23579=DIRECTION('ref_axis',(0.863992480249344,5.75245115886563E-17,0.503504711072882));
#23580=DIRECTION('center_axis',(6.65798752924967E-17,-1.,1.71022579061586E-31));
#23581=DIRECTION('ref_axis',(0.785509852843689,5.22991480433604E-17,0.618849150508818));
#23582=DIRECTION('',(-6.65798752924967E-17,1.,-1.71022579061586E-31));
#23583=DIRECTION('center_axis',(-6.65798752924967E-17,1.,-1.71022579061586E-31));
#23584=DIRECTION('ref_axis',(0.78550985283799,5.22991480429809E-17,0.618849150516052));
#23585=DIRECTION('',(6.65798752924967E-17,-1.,1.71022579061586E-31));
#23586=DIRECTION('center_axis',(6.65798752924967E-17,-1.,1.71022579061586E-31));
#23587=DIRECTION('ref_axis',(0.78550985283799,5.22991480429809E-17,0.618849150516052));
#23588=DIRECTION('center_axis',(6.65798752924967E-17,-1.,1.71022579061586E-31));
#23589=DIRECTION('ref_axis',(0.691738169650181,4.60558410703691E-17,0.72214839517167));
#23590=DIRECTION('',(-6.65798752924967E-17,1.,-1.71022579061586E-31));
#23591=DIRECTION('center_axis',(-6.65798752924967E-17,1.,-1.71022579061586E-31));
#23592=DIRECTION('ref_axis',(0.691738169646283,4.60558410701096E-17,0.722148395175403));
#23593=DIRECTION('',(6.65798752924967E-17,-1.,1.71022579061586E-31));
#23594=DIRECTION('center_axis',(6.65798752924967E-17,-1.,1.71022579061586E-31));
#23595=DIRECTION('ref_axis',(0.691738169646283,4.60558410701096E-17,0.722148395175403));
#23596=DIRECTION('center_axis',(6.65798752924967E-17,-1.,1.71022579061586E-31));
#23597=DIRECTION('ref_axis',(0.584502589824937,3.89161095386858E-17,0.811391842754129));
#23598=DIRECTION('',(-6.65798752924967E-17,1.,-1.71022579061586E-31));
#23599=DIRECTION('center_axis',(-6.65798752924967E-17,1.,-1.71022579061586E-31));
#23600=DIRECTION('ref_axis',(0.584502589823736,3.89161095386059E-17,0.811391842754994));
#23601=DIRECTION('',(6.65798752924967E-17,-1.,1.71022579061586E-31));
#23602=DIRECTION('center_axis',(6.65798752924967E-17,-1.,1.71022579061586E-31));
#23603=DIRECTION('ref_axis',(0.584502589823736,3.89161095386059E-17,0.811391842754994));
#23604=DIRECTION('center_axis',(6.65798752924967E-17,-1.,1.71022579061586E-31));
#23605=DIRECTION('ref_axis',(0.465890331950592,3.10189202012505E-17,0.884842471061921));
#23606=DIRECTION('',(-6.65798752924967E-17,1.,-1.71022579061586E-31));
#23607=DIRECTION('center_axis',(-6.65798752924967E-17,1.,-1.71022579061586E-31));
#23608=DIRECTION('ref_axis',(0.465890331952774,3.10189202013957E-17,0.884842471060773));
#23609=DIRECTION('',(6.65798752924967E-17,-1.,1.71022579061586E-31));
#23610=DIRECTION('center_axis',(6.65798752924967E-17,-1.,1.71022579061586E-31));
#23611=DIRECTION('ref_axis',(0.465890331952774,3.10189202013957E-17,0.884842471060773));
#23612=DIRECTION('center_axis',(6.65798752924967E-17,-1.,1.71022579061586E-31));
#23613=DIRECTION('ref_axis',(0.338210048707227,2.25179828655966E-17,0.941070647163886));
#23614=DIRECTION('',(-6.65798752924967E-17,1.,-1.71022579061586E-31));
#23615=DIRECTION('center_axis',(-6.65798752924967E-17,1.,-1.71022579061586E-31));
#23616=DIRECTION('ref_axis',(0.338210048713215,2.25179828659953E-17,0.941070647161734));
#23617=DIRECTION('',(6.65798752924967E-17,-1.,1.71022579061586E-31));
#23618=DIRECTION('center_axis',(6.65798752924967E-17,-1.,1.71022579061586E-31));
#23619=DIRECTION('ref_axis',(0.338210048713215,2.25179828659953E-17,0.941070647161734));
#23620=DIRECTION('center_axis',(6.65798752924967E-17,-1.,1.71022579061586E-31));
#23621=DIRECTION('ref_axis',(0.203946891574005,1.35787586072898E-17,0.978981953570801));
#23622=DIRECTION('',(-6.65798752924967E-17,1.,-1.71022579061586E-31));
#23623=DIRECTION('center_axis',(-6.65798752924967E-17,1.,-1.71022579061586E-31));
#23624=DIRECTION('ref_axis',(0.203946891583929,1.35787586079505E-17,0.978981953568733));
#23625=DIRECTION('',(6.65798752924967E-17,-1.,1.71022579061586E-31));
#23626=DIRECTION('center_axis',(6.65798752924967E-17,-1.,1.71022579061586E-31));
#23627=DIRECTION('ref_axis',(0.203946891583929,1.35787586079505E-17,0.978981953568733));
#23628=DIRECTION('center_axis',(6.65798752924967E-17,-1.,1.71022579061586E-31));
#23629=DIRECTION('ref_axis',(0.0657141401824452,4.37523925830102E-18,0.997838489826927));
#23630=DIRECTION('',(-6.65798752924967E-17,1.,-1.71022579061586E-31));
#23631=DIRECTION('center_axis',(-6.65798752924967E-17,1.,-1.71022579061586E-31));
#23632=DIRECTION('ref_axis',(0.0657141401961282,4.37523925921203E-18,0.997838489826026));
#23633=DIRECTION('',(6.65798752924967E-17,-1.,1.71022579061586E-31));
#23634=DIRECTION('center_axis',(6.65798752924967E-17,-1.,1.71022579061586E-31));
#23635=DIRECTION('ref_axis',(0.0657141401961282,4.37523925921203E-18,0.997838489826026));
#23636=DIRECTION('center_axis',(6.65798752924967E-17,-1.,1.71022579061586E-31));
#23637=DIRECTION('ref_axis',(-0.0737976621990395,-4.91343914608968E-18,
0.997273234903031));
#23638=DIRECTION('',(-6.65798752924967E-17,1.,-1.71022579061586E-31));
#23639=DIRECTION('center_axis',(-6.65798752924967E-17,1.,-1.71022579061586E-31));
#23640=DIRECTION('ref_axis',(-0.073797662182064,-4.91343914495945E-18,0.997273234904287));
#23641=DIRECTION('',(6.65798752924967E-17,-1.,1.71022579061586E-31));
#23642=DIRECTION('center_axis',(6.65798752924967E-17,-1.,1.71022579061586E-31));
#23643=DIRECTION('ref_axis',(-0.073797662182064,-4.91343914495945E-18,0.997273234904287));
#23644=DIRECTION('center_axis',(6.65798752924967E-17,-1.,1.71022579061586E-31));
#23645=DIRECTION('ref_axis',(0.97729719084324,6.50683250900503E-17,0.211873077029416));
#23646=DIRECTION('center_axis',(-6.65798752924967E-17,1.,-1.71022579061586E-31));
#23647=DIRECTION('ref_axis',(-0.211873077029416,-1.41064830464559E-17,0.97729719084324));
#23648=DIRECTION('center_axis',(6.65798752924967E-17,-1.,1.71022579061586E-31));
#23649=DIRECTION('ref_axis',(-0.211873077029416,-1.41064830464559E-17,0.977297190843239));
#23650=DIRECTION('center_axis',(-6.65798752924967E-17,1.,-1.71022579061586E-31));
#23651=DIRECTION('ref_axis',(-0.211873077029416,-1.41064830464559E-17,0.97729719084324));
#23652=DIRECTION('center_axis',(-6.65798752924967E-17,1.,-1.71022579061586E-31));
#23653=DIRECTION('ref_axis',(-0.211873077029416,-1.41064830464559E-17,0.97729719084324));
#23654=DIRECTION('center_axis',(-6.65798752924967E-17,1.,-1.71022579061586E-31));
#23655=DIRECTION('ref_axis',(-0.211873077029416,-1.41064830464559E-17,0.97729719084324));
#23656=DIRECTION('center_axis',(-6.65798752924967E-17,1.,-1.71022579061586E-31));
#23657=DIRECTION('ref_axis',(-0.211873077029416,-1.41064830464559E-17,0.97729719084324));
#23658=DIRECTION('center_axis',(-6.65798752924967E-17,1.,-1.71022579061586E-31));
#23659=DIRECTION('ref_axis',(-0.211873077029416,-1.41064830464559E-17,0.97729719084324));
#23660=DIRECTION('center_axis',(-6.65798752924967E-17,1.,-1.71022579061586E-31));
#23661=DIRECTION('ref_axis',(-0.211873077029416,-1.41064830464559E-17,0.97729719084324));
#23662=DIRECTION('center_axis',(-6.65798752924967E-17,1.,-1.71022579061586E-31));
#23663=DIRECTION('ref_axis',(-0.211873077029416,-1.41064830464559E-17,0.97729719084324));
#23664=DIRECTION('center_axis',(-6.65798752924967E-17,1.,-1.71022579061586E-31));
#23665=DIRECTION('ref_axis',(-0.211873077029416,-1.41064830464559E-17,0.97729719084324));
#23666=DIRECTION('center_axis',(-6.65798752924967E-17,1.,-1.71022579061586E-31));
#23667=DIRECTION('ref_axis',(-0.211873077029416,-1.41064830464559E-17,0.97729719084324));
#23668=DIRECTION('center_axis',(-6.65798752924967E-17,1.,-1.71022579061586E-31));
#23669=DIRECTION('ref_axis',(-0.211873077029416,-1.41064830464559E-17,0.97729719084324));
#23670=DIRECTION('center_axis',(-6.65798752924967E-17,1.,-1.71022579061586E-31));
#23671=DIRECTION('ref_axis',(-0.211873077029416,-1.41064830464559E-17,0.97729719084324));
#23672=DIRECTION('center_axis',(-6.65798752924967E-17,1.,-1.71022579061586E-31));
#23673=DIRECTION('ref_axis',(-0.211873077029416,-1.41064830464559E-17,0.97729719084324));
#23674=DIRECTION('center_axis',(-6.65798752924967E-17,1.,-1.71022579061586E-31));
#23675=DIRECTION('ref_axis',(-0.211873077029416,-1.41064830464559E-17,0.97729719084324));
#23676=DIRECTION('center_axis',(-6.65798752924967E-17,1.,-1.71022579061586E-31));
#23677=DIRECTION('ref_axis',(-0.211873077029416,-1.41064830464559E-17,0.97729719084324));
#23678=DIRECTION('center_axis',(-6.65798752924967E-17,1.,-1.71022579061586E-31));
#23679=DIRECTION('ref_axis',(-0.211873077029416,-1.41064830464559E-17,0.97729719084324));
#23680=DIRECTION('center_axis',(-6.65798752924967E-17,1.,-1.71022579061586E-31));
#23681=DIRECTION('ref_axis',(-0.211873077029416,-1.41064830464559E-17,0.97729719084324));
#23682=DIRECTION('center_axis',(-6.65798752924967E-17,1.,-1.71022579061586E-31));
#23683=DIRECTION('ref_axis',(-0.211873077029416,-1.41064830464559E-17,0.97729719084324));
#23684=DIRECTION('center_axis',(-6.65798752924967E-17,1.,-1.71022579061586E-31));
#23685=DIRECTION('ref_axis',(-0.211873077029416,-1.41064830464559E-17,0.97729719084324));
#23686=DIRECTION('center_axis',(-6.65798752924967E-17,1.,-1.71022579061586E-31));
#23687=DIRECTION('ref_axis',(-0.211873077029416,-1.41064830464559E-17,0.97729719084324));
#23688=DIRECTION('center_axis',(-6.65798752924967E-17,1.,-1.71022579061586E-31));
#23689=DIRECTION('ref_axis',(-0.211873077029416,-1.41064830464559E-17,0.97729719084324));
#23690=DIRECTION('center_axis',(-6.65798752924967E-17,1.,-1.71022579061586E-31));
#23691=DIRECTION('ref_axis',(-0.211873077029416,-1.41064830464559E-17,0.97729719084324));
#23692=DIRECTION('center_axis',(-6.65798752924967E-17,1.,-1.71022579061586E-31));
#23693=DIRECTION('ref_axis',(-0.211873077029416,-1.41064830464559E-17,0.97729719084324));
#23694=DIRECTION('center_axis',(-6.65798752924967E-17,1.,-1.71022579061586E-31));
#23695=DIRECTION('ref_axis',(-0.211873077029416,-1.41064830464559E-17,0.97729719084324));
#23696=DIRECTION('center_axis',(-6.65798752924967E-17,1.,-1.71022579061586E-31));
#23697=DIRECTION('ref_axis',(-0.211873077029416,-1.41064830464559E-17,0.97729719084324));
#23698=DIRECTION('center_axis',(-6.65798752924967E-17,1.,-1.71022579061586E-31));
#23699=DIRECTION('ref_axis',(-0.211873077029416,-1.41064830464559E-17,0.97729719084324));
#23700=DIRECTION('center_axis',(-6.65798752924967E-17,1.,-1.71022579061586E-31));
#23701=DIRECTION('ref_axis',(-0.211873077029416,-1.41064830464559E-17,0.97729719084324));
#23702=DIRECTION('center_axis',(-6.65798752924967E-17,1.,-1.71022579061586E-31));
#23703=DIRECTION('ref_axis',(-0.211873077029416,-1.41064830464559E-17,0.97729719084324));
#23704=DIRECTION('center_axis',(-6.65798752924967E-17,1.,-1.71022579061586E-31));
#23705=DIRECTION('ref_axis',(-0.211873077029416,-1.41064830464559E-17,0.97729719084324));
#23706=DIRECTION('center_axis',(-6.65798752924967E-17,1.,-1.71022579061586E-31));
#23707=DIRECTION('ref_axis',(-0.211873077029416,-1.41064830464559E-17,0.97729719084324));
#23708=DIRECTION('center_axis',(-6.65798752924967E-17,1.,-1.71022579061586E-31));
#23709=DIRECTION('ref_axis',(-0.211873077029416,-1.41064830464559E-17,0.97729719084324));
#23710=DIRECTION('center_axis',(-6.65798752924967E-17,1.,-1.71022579061586E-31));
#23711=DIRECTION('ref_axis',(-0.211873077029416,-1.41064830464559E-17,0.97729719084324));
#23712=DIRECTION('center_axis',(-6.65798752924967E-17,1.,-1.71022579061586E-31));
#23713=DIRECTION('ref_axis',(-0.211873077029416,-1.41064830464559E-17,0.97729719084324));
#23714=DIRECTION('center_axis',(-6.65798752924967E-17,1.,-1.71022579061586E-31));
#23715=DIRECTION('ref_axis',(-0.211873077029416,-1.41064830464559E-17,0.97729719084324));
#23716=DIRECTION('center_axis',(-6.65798752924967E-17,1.,-1.71022579061586E-31));
#23717=DIRECTION('ref_axis',(-0.211873077029416,-1.41064830464559E-17,0.97729719084324));
#23718=DIRECTION('center_axis',(-6.65798752924967E-17,1.,-1.71022579061586E-31));
#23719=DIRECTION('ref_axis',(-0.211873077029416,-1.41064830464559E-17,0.97729719084324));
#23720=DIRECTION('center_axis',(-6.65798752924967E-17,1.,-1.71022579061586E-31));
#23721=DIRECTION('ref_axis',(-0.211873077029416,-1.41064830464559E-17,0.97729719084324));
#23722=DIRECTION('center_axis',(-6.65798752924967E-17,1.,-1.71022579061586E-31));
#23723=DIRECTION('ref_axis',(-0.211873077029416,-1.41064830464559E-17,0.97729719084324));
#23724=DIRECTION('center_axis',(-6.65798752924967E-17,1.,-1.71022579061586E-31));
#23725=DIRECTION('ref_axis',(-0.211873077029416,-1.41064830464559E-17,0.97729719084324));
#23726=DIRECTION('center_axis',(-6.65798752924967E-17,1.,-1.71022579061586E-31));
#23727=DIRECTION('ref_axis',(-0.211873077029416,-1.41064830464559E-17,0.97729719084324));
#23728=DIRECTION('center_axis',(-6.65798752924967E-17,1.,-1.71022579061586E-31));
#23729=DIRECTION('ref_axis',(-0.211873077029416,-1.41064830464559E-17,0.97729719084324));
#23730=DIRECTION('center_axis',(-6.65798752924967E-17,1.,-1.71022579061586E-31));
#23731=DIRECTION('ref_axis',(-0.211873077029416,-1.41064830464559E-17,0.97729719084324));
#23732=DIRECTION('center_axis',(-6.65798752924967E-17,1.,-1.71022579061586E-31));
#23733=DIRECTION('ref_axis',(-0.211873077029416,-1.41064830464559E-17,0.97729719084324));
#23734=DIRECTION('center_axis',(-6.65798752924967E-17,1.,-1.71022579061586E-31));
#23735=DIRECTION('ref_axis',(-0.211873077029416,-1.41064830464559E-17,0.97729719084324));
#23736=DIRECTION('center_axis',(-6.65798752924967E-17,1.,-1.71022579061586E-31));
#23737=DIRECTION('ref_axis',(-0.211873077029416,-1.41064830464559E-17,0.97729719084324));
#23738=DIRECTION('center_axis',(6.65798752924967E-17,-1.,1.71022579061586E-31));
#23739=DIRECTION('ref_axis',(0.211873077029416,1.41064830464559E-17,-0.977297190843239));
#23740=DIRECTION('center_axis',(-6.65798752924967E-17,1.,-1.71022579061586E-31));
#23741=DIRECTION('ref_axis',(-0.211873077029416,-1.41064830464559E-17,0.977297190843239));
#23742=DIRECTION('center_axis',(6.65798752924967E-17,-1.,1.71022579061586E-31));
#23743=DIRECTION('ref_axis',(-0.211873077029416,-1.41064830464559E-17,0.97729719084324));
#23744=DIRECTION('',(-6.65798752924967E-17,1.,-1.71022579061586E-31));
#23745=DIRECTION('center_axis',(-6.65798752924967E-17,1.,-1.71022579061586E-31));
#23746=DIRECTION('ref_axis',(-0.211873077029416,-1.41064830464559E-17,0.977297190843239));
#23747=DIRECTION('',(6.65798752924967E-17,-1.,1.71022579061586E-31));
#23748=DIRECTION('center_axis',(6.65798752924967E-17,-1.,1.71022579061586E-31));
#23749=DIRECTION('ref_axis',(-0.211873077029416,-1.41064830464559E-17,0.97729719084324));
#23750=DIRECTION('center_axis',(-6.65798752924967E-17,1.,-1.71022579061586E-31));
#23751=DIRECTION('ref_axis',(-0.211873077029416,-1.41064830464559E-17,0.977297190843239));
#23752=DIRECTION('center_axis',(6.65798752924967E-17,-1.,1.71022579061586E-31));
#23753=DIRECTION('ref_axis',(-0.211873077029416,-1.41064830464559E-17,0.97729719084324));
#23754=DIRECTION('center_axis',(-6.65798752924967E-17,1.,-1.71022579061586E-31));
#23755=DIRECTION('ref_axis',(-0.211873077029416,-1.41064830464559E-17,0.977297190843239));
#23756=DIRECTION('center_axis',(6.65798752924967E-17,-1.,1.71022579061586E-31));
#23757=DIRECTION('ref_axis',(-0.211873077029416,-1.41064830464559E-17,0.97729719084324));
#23758=DIRECTION('center_axis',(-6.65798752924967E-17,1.,-1.71022579061586E-31));
#23759=DIRECTION('ref_axis',(-0.211873077029416,-1.41064830464559E-17,0.977297190843239));
#23760=DIRECTION('center_axis',(6.65798752924967E-17,-1.,1.71022579061586E-31));
#23761=DIRECTION('ref_axis',(-0.211873077029416,-1.41064830464559E-17,0.97729719084324));
#23762=DIRECTION('center_axis',(-6.65798752924967E-17,1.,-1.71022579061586E-31));
#23763=DIRECTION('ref_axis',(-0.211873077029416,-1.41064830464559E-17,0.977297190843239));
#23764=DIRECTION('center_axis',(6.65798752924967E-17,-1.,1.71022579061586E-31));
#23765=DIRECTION('ref_axis',(-0.211873077029416,-1.41064830464559E-17,0.97729719084324));
#23766=DIRECTION('center_axis',(-6.65798752924967E-17,1.,-1.71022579061586E-31));
#23767=DIRECTION('ref_axis',(-0.211873077029416,-1.41064830464559E-17,0.977297190843239));
#23768=DIRECTION('center_axis',(6.65798752924967E-17,-1.,1.71022579061586E-31));
#23769=DIRECTION('ref_axis',(-0.211873077029416,-1.41064830464559E-17,0.97729719084324));
#23770=DIRECTION('center_axis',(-6.65798752924967E-17,1.,-1.71022579061586E-31));
#23771=DIRECTION('ref_axis',(-0.211873077029416,-1.41064830464559E-17,0.977297190843239));
#23772=DIRECTION('center_axis',(6.65798752924967E-17,-1.,1.71022579061586E-31));
#23773=DIRECTION('ref_axis',(-0.211873077029416,-1.41064830464559E-17,0.97729719084324));
#23774=DIRECTION('center_axis',(-6.65798752924967E-17,1.,-1.71022579061586E-31));
#23775=DIRECTION('ref_axis',(-0.211873077029416,-1.41064830464559E-17,0.977297190843239));
#23776=DIRECTION('center_axis',(6.65798752924967E-17,-1.,1.71022579061586E-31));
#23777=DIRECTION('ref_axis',(-0.211873077029416,-1.41064830464559E-17,0.97729719084324));
#23778=DIRECTION('center_axis',(-6.65798752924967E-17,1.,-1.71022579061586E-31));
#23779=DIRECTION('ref_axis',(-0.211873077029416,-1.41064830464559E-17,0.977297190843239));
#23780=DIRECTION('center_axis',(6.65798752924967E-17,-1.,1.71022579061586E-31));
#23781=DIRECTION('ref_axis',(-0.211873077029416,-1.41064830464559E-17,0.97729719084324));
#23782=DIRECTION('center_axis',(-6.65798752924967E-17,1.,-1.71022579061586E-31));
#23783=DIRECTION('ref_axis',(-0.211873077029416,-1.41064830464559E-17,0.977297190843239));
#23784=DIRECTION('center_axis',(6.65798752924967E-17,-1.,1.71022579061586E-31));
#23785=DIRECTION('ref_axis',(-0.211873077029416,-1.41064830464559E-17,0.97729719084324));
#23786=DIRECTION('center_axis',(-6.65798752924967E-17,1.,-1.71022579061586E-31));
#23787=DIRECTION('ref_axis',(-0.211873077029416,-1.41064830464559E-17,0.977297190843239));
#23788=DIRECTION('center_axis',(6.65798752924967E-17,-1.,1.71022579061586E-31));
#23789=DIRECTION('ref_axis',(-0.211873077029416,-1.41064830464559E-17,0.97729719084324));
#23790=DIRECTION('center_axis',(-6.65798752924967E-17,1.,-1.71022579061586E-31));
#23791=DIRECTION('ref_axis',(-0.211873077029416,-1.41064830464559E-17,0.977297190843239));
#23792=DIRECTION('center_axis',(6.65798752924967E-17,-1.,1.71022579061586E-31));
#23793=DIRECTION('ref_axis',(-0.211873077029416,-1.41064830464559E-17,0.97729719084324));
#23794=DIRECTION('center_axis',(-6.65798752924967E-17,1.,-1.71022579061586E-31));
#23795=DIRECTION('ref_axis',(-0.211873077029416,-1.41064830464559E-17,0.977297190843239));
#23796=DIRECTION('center_axis',(6.65798752924967E-17,-1.,1.71022579061586E-31));
#23797=DIRECTION('ref_axis',(-0.211873077029416,-1.41064830464559E-17,0.97729719084324));
#23798=DIRECTION('center_axis',(-6.65798752924967E-17,1.,-1.71022579061586E-31));
#23799=DIRECTION('ref_axis',(-0.211873077029416,-1.41064830464559E-17,0.977297190843239));
#23800=DIRECTION('center_axis',(6.65798752924967E-17,-1.,1.71022579061586E-31));
#23801=DIRECTION('ref_axis',(-0.211873077029416,-1.41064830464559E-17,0.97729719084324));
#23802=DIRECTION('center_axis',(-6.65798752924967E-17,1.,-1.71022579061586E-31));
#23803=DIRECTION('ref_axis',(-0.211873077029416,-1.41064830464559E-17,0.977297190843239));
#23804=DIRECTION('center_axis',(6.65798752924967E-17,-1.,1.71022579061586E-31));
#23805=DIRECTION('ref_axis',(-0.211873077029416,-1.41064830464559E-17,0.97729719084324));
#23806=DIRECTION('center_axis',(-6.65798752924967E-17,1.,-1.71022579061586E-31));
#23807=DIRECTION('ref_axis',(-0.211873077029416,-1.41064830464559E-17,0.977297190843239));
#23808=DIRECTION('center_axis',(6.65798752924967E-17,-1.,1.71022579061586E-31));
#23809=DIRECTION('ref_axis',(-0.211873077029416,-1.41064830464559E-17,0.97729719084324));
#23810=DIRECTION('center_axis',(-6.65798752924967E-17,1.,-1.71022579061586E-31));
#23811=DIRECTION('ref_axis',(-0.211873077029416,-1.41064830464559E-17,0.977297190843239));
#23812=DIRECTION('center_axis',(6.65798752924967E-17,-1.,1.71022579061586E-31));
#23813=DIRECTION('ref_axis',(-0.211873077029416,-1.41064830464559E-17,0.97729719084324));
#23814=DIRECTION('center_axis',(-6.65798752924967E-17,1.,-1.71022579061586E-31));
#23815=DIRECTION('ref_axis',(-0.211873077029416,-1.41064830464559E-17,0.977297190843239));
#23816=DIRECTION('center_axis',(6.65798752924967E-17,-1.,1.71022579061586E-31));
#23817=DIRECTION('ref_axis',(-0.211873077029416,-1.41064830464559E-17,0.97729719084324));
#23818=DIRECTION('center_axis',(-6.65798752924967E-17,1.,-1.71022579061586E-31));
#23819=DIRECTION('ref_axis',(-0.211873077029416,-1.41064830464559E-17,0.977297190843239));
#23820=DIRECTION('center_axis',(6.65798752924967E-17,-1.,1.71022579061586E-31));
#23821=DIRECTION('ref_axis',(-0.211873077029416,-1.41064830464559E-17,0.97729719084324));
#23822=DIRECTION('center_axis',(-6.65798752924967E-17,1.,-1.71022579061586E-31));
#23823=DIRECTION('ref_axis',(-0.211873077029416,-1.41064830464559E-17,0.977297190843239));
#23824=DIRECTION('center_axis',(6.65798752924967E-17,-1.,1.71022579061586E-31));
#23825=DIRECTION('ref_axis',(-0.211873077029416,-1.41064830464559E-17,0.97729719084324));
#23826=DIRECTION('center_axis',(-6.65798752924967E-17,1.,-1.71022579061586E-31));
#23827=DIRECTION('ref_axis',(-0.211873077029416,-1.41064830464559E-17,0.977297190843239));
#23828=DIRECTION('center_axis',(6.65798752924967E-17,-1.,1.71022579061586E-31));
#23829=DIRECTION('ref_axis',(-0.211873077029416,-1.41064830464559E-17,0.97729719084324));
#23830=DIRECTION('center_axis',(-6.65798752924967E-17,1.,-1.71022579061586E-31));
#23831=DIRECTION('ref_axis',(-0.211873077029416,-1.41064830464559E-17,0.977297190843239));
#23832=DIRECTION('center_axis',(6.65798752924967E-17,-1.,1.71022579061586E-31));
#23833=DIRECTION('ref_axis',(-0.211873077029416,-1.41064830464559E-17,0.97729719084324));
#23834=DIRECTION('center_axis',(-6.65798752924967E-17,1.,-1.71022579061586E-31));
#23835=DIRECTION('ref_axis',(-0.211873077029416,-1.41064830464559E-17,0.977297190843239));
#23836=DIRECTION('center_axis',(6.65798752924967E-17,-1.,1.71022579061586E-31));
#23837=DIRECTION('ref_axis',(-0.211873077029416,-1.41064830464559E-17,0.97729719084324));
#23838=DIRECTION('center_axis',(-6.65798752924967E-17,1.,-1.71022579061586E-31));
#23839=DIRECTION('ref_axis',(-0.211873077029416,-1.41064830464559E-17,0.977297190843239));
#23840=DIRECTION('center_axis',(6.65798752924967E-17,-1.,1.71022579061586E-31));
#23841=DIRECTION('ref_axis',(-0.211873077029416,-1.41064830464559E-17,0.97729719084324));
#23842=DIRECTION('center_axis',(-6.65798752924967E-17,1.,-1.71022579061586E-31));
#23843=DIRECTION('ref_axis',(-0.211873077029416,-1.41064830464559E-17,0.977297190843239));
#23844=DIRECTION('center_axis',(6.65798752924967E-17,-1.,1.71022579061586E-31));
#23845=DIRECTION('ref_axis',(-0.211873077029416,-1.41064830464559E-17,0.97729719084324));
#23846=DIRECTION('center_axis',(-6.65798752924967E-17,1.,-1.71022579061586E-31));
#23847=DIRECTION('ref_axis',(-0.211873077029416,-1.41064830464559E-17,0.977297190843239));
#23848=DIRECTION('center_axis',(6.65798752924967E-17,-1.,1.71022579061586E-31));
#23849=DIRECTION('ref_axis',(-0.211873077029416,-1.41064830464559E-17,0.97729719084324));
#23850=DIRECTION('center_axis',(-6.65798752924967E-17,1.,-1.71022579061586E-31));
#23851=DIRECTION('ref_axis',(-0.211873077029416,-1.41064830464559E-17,0.977297190843239));
#23852=DIRECTION('center_axis',(6.65798752924967E-17,-1.,1.71022579061586E-31));
#23853=DIRECTION('ref_axis',(-0.211873077029416,-1.41064830464559E-17,0.97729719084324));
#23854=DIRECTION('center_axis',(-6.65798752924967E-17,1.,-1.71022579061586E-31));
#23855=DIRECTION('ref_axis',(-0.211873077029416,-1.41064830464559E-17,0.977297190843239));
#23856=DIRECTION('center_axis',(6.65798752924967E-17,-1.,1.71022579061586E-31));
#23857=DIRECTION('ref_axis',(-0.211873077029416,-1.41064830464559E-17,0.97729719084324));
#23858=DIRECTION('center_axis',(-6.65798752924967E-17,1.,-1.71022579061586E-31));
#23859=DIRECTION('ref_axis',(-0.211873077029416,-1.41064830464559E-17,0.977297190843239));
#23860=DIRECTION('center_axis',(6.65798752924967E-17,-1.,1.71022579061586E-31));
#23861=DIRECTION('ref_axis',(-0.211873077029416,-1.41064830464559E-17,0.97729719084324));
#23862=DIRECTION('center_axis',(-6.65798752924967E-17,1.,-1.71022579061586E-31));
#23863=DIRECTION('ref_axis',(-0.211873077029416,-1.41064830464559E-17,0.977297190843239));
#23864=DIRECTION('center_axis',(6.65798752924967E-17,-1.,1.71022579061586E-31));
#23865=DIRECTION('ref_axis',(-0.211873077029416,-1.41064830464559E-17,0.97729719084324));
#23866=DIRECTION('center_axis',(-6.65798752924967E-17,1.,-1.71022579061586E-31));
#23867=DIRECTION('ref_axis',(-0.211873077029416,-1.41064830464559E-17,0.977297190843239));
#23868=DIRECTION('center_axis',(6.65798752924967E-17,-1.,1.71022579061586E-31));
#23869=DIRECTION('ref_axis',(-0.211873077029416,-1.41064830464559E-17,0.97729719084324));
#23870=DIRECTION('center_axis',(-6.65798752924967E-17,1.,-1.71022579061586E-31));
#23871=DIRECTION('ref_axis',(-0.211873077029416,-1.41064830464559E-17,0.977297190843239));
#23872=DIRECTION('center_axis',(6.65798752924967E-17,-1.,1.71022579061586E-31));
#23873=DIRECTION('ref_axis',(-0.211873077029416,-1.41064830464559E-17,0.97729719084324));
#23874=DIRECTION('center_axis',(-6.65798752924967E-17,1.,-1.71022579061586E-31));
#23875=DIRECTION('ref_axis',(-0.211873077029416,-1.41064830464559E-17,0.977297190843239));
#23876=DIRECTION('center_axis',(6.65798752924967E-17,-1.,1.71022579061586E-31));
#23877=DIRECTION('ref_axis',(-0.211873077029416,-1.41064830464559E-17,0.97729719084324));
#23878=DIRECTION('center_axis',(-6.65798752924967E-17,1.,-1.71022579061586E-31));
#23879=DIRECTION('ref_axis',(-0.211873077029416,-1.41064830464559E-17,0.977297190843239));
#23880=DIRECTION('center_axis',(6.65798752924967E-17,-1.,1.71022579061586E-31));
#23881=DIRECTION('ref_axis',(-0.211873077029416,-1.41064830464559E-17,0.97729719084324));
#23882=DIRECTION('center_axis',(-6.65798752924967E-17,1.,-1.71022579061586E-31));
#23883=DIRECTION('ref_axis',(-0.211873077029416,-1.41064830464559E-17,0.977297190843239));
#23884=DIRECTION('center_axis',(6.65798752924967E-17,-1.,1.71022579061586E-31));
#23885=DIRECTION('ref_axis',(-0.211873077029416,-1.41064830464559E-17,0.97729719084324));
#23886=DIRECTION('center_axis',(-6.65798752924967E-17,1.,-1.71022579061586E-31));
#23887=DIRECTION('ref_axis',(-0.211873077029416,-1.41064830464559E-17,0.977297190843239));
#23888=DIRECTION('center_axis',(6.65798752924967E-17,-1.,1.71022579061586E-31));
#23889=DIRECTION('ref_axis',(-0.211873077029416,-1.41064830464559E-17,0.97729719084324));
#23890=DIRECTION('center_axis',(-6.65798752924967E-17,1.,-1.71022579061586E-31));
#23891=DIRECTION('ref_axis',(-0.211873077029416,-1.41064830464559E-17,0.977297190843239));
#23892=DIRECTION('center_axis',(6.65798752924967E-17,-1.,1.71022579061586E-31));
#23893=DIRECTION('ref_axis',(-0.211873077029416,-1.41064830464559E-17,0.97729719084324));
#23894=DIRECTION('center_axis',(-6.65798752924967E-17,1.,-1.71022579061586E-31));
#23895=DIRECTION('ref_axis',(-0.211873077029416,-1.41064830464559E-17,0.977297190843239));
#23896=DIRECTION('center_axis',(6.65798752924967E-17,-1.,1.71022579061586E-31));
#23897=DIRECTION('ref_axis',(-0.211873077029416,-1.41064830464559E-17,0.97729719084324));
#23898=DIRECTION('center_axis',(-6.65798752924967E-17,1.,-1.71022579061586E-31));
#23899=DIRECTION('ref_axis',(-0.211873077029416,-1.41064830464559E-17,0.977297190843239));
#23900=DIRECTION('center_axis',(6.65798752924967E-17,-1.,1.71022579061586E-31));
#23901=DIRECTION('ref_axis',(-0.211873077029416,-1.41064830464559E-17,0.97729719084324));
#23902=DIRECTION('center_axis',(-6.65798752924967E-17,1.,-1.71022579061586E-31));
#23903=DIRECTION('ref_axis',(-0.211873077029416,-1.41064830464559E-17,0.977297190843239));
#23904=DIRECTION('center_axis',(6.65798752924967E-17,-1.,1.71022579061586E-31));
#23905=DIRECTION('ref_axis',(-0.211873077029416,-1.41064830464559E-17,0.97729719084324));
#23906=DIRECTION('center_axis',(-6.65798752924967E-17,1.,-1.71022579061586E-31));
#23907=DIRECTION('ref_axis',(-0.211873077029416,-1.41064830464559E-17,0.977297190843239));
#23908=DIRECTION('center_axis',(6.65798752924967E-17,-1.,1.71022579061586E-31));
#23909=DIRECTION('ref_axis',(-0.211873077029416,-1.41064830464559E-17,0.97729719084324));
#23910=DIRECTION('center_axis',(-6.65798752924967E-17,1.,-1.71022579061586E-31));
#23911=DIRECTION('ref_axis',(-0.211873077029416,-1.41064830464559E-17,0.977297190843239));
#23912=DIRECTION('center_axis',(6.65798752924967E-17,-1.,1.71022579061586E-31));
#23913=DIRECTION('ref_axis',(-0.211873077029416,-1.41064830464559E-17,0.97729719084324));
#23914=DIRECTION('center_axis',(-6.65798752924967E-17,1.,-1.71022579061586E-31));
#23915=DIRECTION('ref_axis',(-0.211873077029416,-1.41064830464559E-17,0.977297190843239));
#23916=DIRECTION('center_axis',(6.65798752924967E-17,-1.,1.71022579061586E-31));
#23917=DIRECTION('ref_axis',(-0.211873077029416,-1.41064830464559E-17,0.97729719084324));
#23918=DIRECTION('center_axis',(6.65798752924967E-17,-1.,1.71022579061586E-31));
#23919=DIRECTION('ref_axis',(-0.211873077029416,-1.41064830464559E-17,0.977297190843239));
#23920=DIRECTION('center_axis',(-6.65798752924967E-17,1.,-1.71022579061586E-31));
#23921=DIRECTION('ref_axis',(-0.211873077029416,-1.41064830464559E-17,0.977297190843239));
#23922=DIRECTION('center_axis',(6.65798752924967E-17,-1.,1.71022579061586E-31));
#23923=DIRECTION('ref_axis',(0.97729719084324,6.50683250900503E-17,0.211873077029416));
#23924=DIRECTION('center_axis',(6.65798752924967E-17,-1.,1.71022579061586E-31));
#23925=DIRECTION('ref_axis',(-0.211873077029416,-1.41064830464559E-17,0.97729719084324));
#23926=DIRECTION('center_axis',(-6.65798752924967E-17,1.,-1.71022579061586E-31));
#23927=DIRECTION('ref_axis',(0.211873077029416,1.41064830464559E-17,-0.977297190843239));
#23928=DIRECTION('center_axis',(-6.65798752924967E-17,1.,-1.71022579061586E-31));
#23929=DIRECTION('ref_axis',(-0.211873077029416,-1.41064830464559E-17,0.977297190843239));
#23930=DIRECTION('center_axis',(-6.65798752924967E-17,1.,-1.71022579061586E-31));
#23931=DIRECTION('ref_axis',(0.211873077029416,1.41064830464559E-17,-0.97729719084324));
#23932=DIRECTION('',(-6.65798752924967E-17,1.,-1.71022579061586E-31));
#29753=CARTESIAN_POINT('',(0.,0.,0.));
#29754=CARTESIAN_POINT('Origin',(0.0121040592752336,-0.01,0.00446113764208535));
#29755=CARTESIAN_POINT('',(0.0119220873914306,-0.0225,0.0049268481031072));
#29756=CARTESIAN_POINT('',(0.0119220873914306,-0.017,0.0049268481031072));
#29757=CARTESIAN_POINT('',(0.0119220873914382,-0.01000000000001,0.00492684810311909));
#29758=CARTESIAN_POINT('',(0.0122678470666214,-0.0225,0.00398872515347788));
#29759=CARTESIAN_POINT('Origin',(0.0121040592752413,-0.02250000000001,0.00446113764209724));
#29760=CARTESIAN_POINT('',(0.0122678470666214,-0.017,0.00398872515347788));
#29761=CARTESIAN_POINT('',(0.0122678470666291,-0.01000000000001,0.00398872515348977));
#29762=CARTESIAN_POINT('Origin',(0.0121040592752413,-0.01700000000001,0.00446113764209724));
#29763=CARTESIAN_POINT('Origin',(0.0113653930429603,-0.01,0.00610228162075688));
#29764=CARTESIAN_POINT('',(0.0111203777280115,-0.0225,0.00653813422822932));
#29765=CARTESIAN_POINT('',(0.0111203777280115,-0.017,0.00653813422822932));
#29766=CARTESIAN_POINT('',(0.0111203777280192,-0.01000000000001,0.00653813422824121));
#29767=CARTESIAN_POINT('',(0.0115933339737932,-0.0225,0.00565726147284101));
#29768=CARTESIAN_POINT('Origin',(0.011365393042968,-0.02250000000001,0.00610228162076877));
#29769=CARTESIAN_POINT('',(0.0115933339737932,-0.017,0.00565726147284101));
#29770=CARTESIAN_POINT('',(0.0115933339738008,-0.01000000000001,0.0056572614728529));
#29771=CARTESIAN_POINT('Origin',(0.011365393042968,-0.01700000000001,0.00610228162076877));
#29772=CARTESIAN_POINT('Origin',(0.0104055123630489,-0.01,0.00762465162892286));
#29773=CARTESIAN_POINT('',(0.010102222561359,-0.0225,0.00802216300761644));
#29774=CARTESIAN_POINT('',(0.010102222561359,-0.017,0.00802216300761644));
#29775=CARTESIAN_POINT('',(0.0101022225613666,-0.01000000000001,0.00802216300762832));
#29776=CARTESIAN_POINT('',(0.0106931698223871,-0.0225,0.00721568563267486));
#29777=CARTESIAN_POINT('Origin',(0.0104055123630566,-0.02250000000001,0.00762465162893475));
#29778=CARTESIAN_POINT('',(0.0106931698223871,-0.017,0.00721568563267486));
#29779=CARTESIAN_POINT('',(0.0106931698223947,-0.01000000000001,0.00721568563268675));
#29780=CARTESIAN_POINT('Origin',(0.0104055123630566,-0.01700000000001,0.00762465162893475));
#29781=CARTESIAN_POINT('Origin',(0.00924310022108555,-0.01,0.00899861646604452));
#29782=CARTESIAN_POINT('',(0.00888743912365737,-0.0225,0.00935004950913547));
#29783=CARTESIAN_POINT('',(0.00888743912365737,-0.017,0.00935004950913547));
#29784=CARTESIAN_POINT('',(0.00888743912366502,-0.01000000000001,0.00935004950914736));
#29785=CARTESIAN_POINT('',(0.00958487528368847,-0.0225,0.00863366467938941));
#29786=CARTESIAN_POINT('Origin',(0.00924310022109321,-0.02250000000001,
0.00899861646605642));
#29787=CARTESIAN_POINT('',(0.00958487528368847,-0.017,0.00863366467938941));
#29788=CARTESIAN_POINT('',(0.00958487528369612,-0.01000000000001,0.00863366467940131));
#29789=CARTESIAN_POINT('Origin',(0.00924310022109321,-0.01700000000001,
0.00899861646605642));
#29790=CARTESIAN_POINT('Origin',(0.00790078164718944,-0.01,0.0101974334694291));
#29791=CARTESIAN_POINT('',(0.0074996717927259,-0.0225,0.0104959479324828));
#29792=CARTESIAN_POINT('',(0.0074996717927259,-0.017,0.0104959479324828));
#29793=CARTESIAN_POINT('',(0.00749967179273355,-0.01000000000001,0.0104959479324947));
#29794=CARTESIAN_POINT('',(0.00829002205022697,-0.0225,0.00988359926376768));
#29795=CARTESIAN_POINT('Origin',(0.0079007816471971,-0.02250000000001,0.010197433469441));
#29796=CARTESIAN_POINT('',(0.00829002205022697,-0.017,0.00988359926376768));
#29797=CARTESIAN_POINT('',(0.00829002205023463,-0.01000000000001,0.00988359926377957));
#29798=CARTESIAN_POINT('Origin',(0.0079007816471971,-0.01700000000001,0.010197433469441));
#29799=CARTESIAN_POINT('Origin',(0.00640468334553672,-0.01,0.01119776902974));
#29800=CARTESIAN_POINT('',(0.00596593188109928,-0.0225,0.0114375546682883));
#29801=CARTESIAN_POINT('',(0.00596593188109928,-0.017,0.0114375546682883));
#29802=CARTESIAN_POINT('',(0.00596593188110694,-0.01000000000001,0.0114375546683002));
#29803=CARTESIAN_POINT('',(0.00683381296731816,-0.0225,0.0109411608309043));
#29804=CARTESIAN_POINT('Origin',(0.00640468334554438,-0.02250000000001,
0.0111977690297519));
#29805=CARTESIAN_POINT('',(0.00683381296731816,-0.017,0.0109411608309043));
#29806=CARTESIAN_POINT('',(0.00683381296732582,-0.01000000000001,0.0109411608309161));
#29807=CARTESIAN_POINT('Origin',(0.00640468334554438,-0.01700000000001,
0.0111977690297519));
#29808=CARTESIAN_POINT('Origin',(0.00478392516778247,-0.01,0.0119801527531604));
#29809=CARTESIAN_POINT('',(0.004316071891554,-0.0225,0.0121565424125011));
#29810=CARTESIAN_POINT('',(0.004316071891554,-0.017,0.0121565424125011));
#29811=CARTESIAN_POINT('',(0.00431607189156165,-0.01000000000001,0.012156542412513));
#29812=CARTESIAN_POINT('',(0.00524459148834751,-0.0225,0.0117857651478533));
#29813=CARTESIAN_POINT('Origin',(0.00478392516779012,-0.02250000000001,
0.0119801527531723));
#29814=CARTESIAN_POINT('',(0.00524459148834751,-0.017,0.0117857651478533));
#29815=CARTESIAN_POINT('',(0.00524459148835515,-0.01000000000001,0.0117857651478652));
#29816=CARTESIAN_POINT('Origin',(0.00478392516779012,-0.01700000000001,
0.0119801527531723));
#29817=CARTESIAN_POINT('Origin',(0.00307005332827152,-0.01,0.0125293564304624));
#29818=CARTESIAN_POINT('',(0.00258220447209863,-0.0225,0.0126389168865166));
#29819=CARTESIAN_POINT('',(0.00258220447209863,-0.017,0.0126389168865166));
#29820=CARTESIAN_POINT('',(0.00258220447210628,-0.01000000000001,0.0126389168865285));
#29821=CARTESIAN_POINT('',(0.00355329000169056,-0.0225,0.0124009729523085));
#29822=CARTESIAN_POINT('Origin',(0.00307005332827917,-0.02250000000001,
0.0125293564304743));
#29823=CARTESIAN_POINT('',(0.00355329000169056,-0.017,0.0124009729523085));
#29824=CARTESIAN_POINT('',(0.00355329000169822,-0.01000000000001,0.0124009729523203));
#29825=CARTESIAN_POINT('Origin',(0.00307005332827917,-0.01700000000001,
0.0125293564304743));
#29826=CARTESIAN_POINT('Origin',(0.00129642639285968,-0.01,0.0128346904367771));
#29827=CARTESIAN_POINT('',(0.000798077379807919,-0.0225,0.0128752892198909));
#29828=CARTESIAN_POINT('',(0.000798077379807918,-0.017,0.0128752892198909));
#29829=CARTESIAN_POINT('',(0.000798077379815572,-0.01000000000001,0.0128752892199028));
#29830=CARTESIAN_POINT('',(0.00179282776695818,-0.0225,0.0127748099241446));
#29831=CARTESIAN_POINT('Origin',(0.00129642639286733,-0.02250000000001,
0.012834690436789));
#29832=CARTESIAN_POINT('',(0.00179282776695818,-0.017,0.0127748099241446));
#29833=CARTESIAN_POINT('',(0.00179282776696584,-0.01000000000001,0.0127748099241565));
#29834=CARTESIAN_POINT('Origin',(0.00129642639286733,-0.01700000000001,
0.012834690436789));
#29835=CARTESIAN_POINT('Origin',(-0.000502434007626007,-0.01,0.0128902117929839));
#29836=CARTESIAN_POINT('',(-0.00100158338088122,-0.0225,0.0128610586940245));
#29837=CARTESIAN_POINT('',(-0.00100158338088122,-0.017,0.0128610586940245));
#29838=CARTESIAN_POINT('',(-0.00100158338087356,-0.01000000000001,0.0128610586940364));
#29839=CARTESIAN_POINT('',(-2.52982094668671E-6,-0.0225,0.0128999997519382));
#29840=CARTESIAN_POINT('Origin',(-0.000502434007618352,-0.02250000000001,
0.0128902117929958));
#29841=CARTESIAN_POINT('',(-2.52982094668715E-6,-0.017,0.0128999997519382));
#29842=CARTESIAN_POINT('',(-2.52982093903355E-6,-0.01000000000001,0.0128999997519501));
#29843=CARTESIAN_POINT('Origin',(-0.000502434007618352,-0.01700000000001,
0.0128902117929958));
#29844=CARTESIAN_POINT('Origin',(-0.00229151510166345,-0.01,0.0126948398390388));
#29845=CARTESIAN_POINT('',(-0.00278174946034568,-0.0225,0.0125965022899163));
#29846=CARTESIAN_POINT('',(-0.00278174946034568,-0.017,0.0125965022899163));
#29847=CARTESIAN_POINT('',(-0.00278174946035758,-0.01000000000001,0.012596502289924));
#29848=CARTESIAN_POINT('',(-0.00179783816876445,-0.0225,0.0127741057580926));
#29849=CARTESIAN_POINT('Origin',(-0.00229151510165579,-0.02250000000001,
0.0126948398390507));
#29850=CARTESIAN_POINT('',(-0.00179783816876445,-0.017,0.0127741057580926));
#29851=CARTESIAN_POINT('',(-0.0017978381687568,-0.01000000000001,0.0127741057581045));
#29852=CARTESIAN_POINT('Origin',(-0.00229151510165579,-0.01700000000001,
0.0126948398390507));
#29853=CARTESIAN_POINT('Origin',(-0.00403599446080683,-0.01,0.0122523772677932));
#29854=CARTESIAN_POINT('',(-0.00450777195075764,-0.0225,0.0120867692970439));
#29855=CARTESIAN_POINT('',(-0.00450777195075764,-0.017,0.0120867692970439));
#29856=CARTESIAN_POINT('',(-0.00450777195076953,-0.01000000000001,0.0120867692970515));
#29857=CARTESIAN_POINT('',(-0.00355815364163782,-0.0225,0.0123995783259956));
#29858=CARTESIAN_POINT('Origin',(-0.00403599446081873,-0.02250000000001,
0.0122523772678009));
#29859=CARTESIAN_POINT('',(-0.00355815364163782,-0.017,0.0123995783259956));
#29860=CARTESIAN_POINT('',(-0.00355815364164971,-0.01000000000001,0.0123995783260032));
#29861=CARTESIAN_POINT('Origin',(-0.00403599446081873,-0.01700000000001,
0.0122523772678009));
#29862=CARTESIAN_POINT('Origin',(-0.00570191777864627,-0.01,0.0115714361099027));
#29863=CARTESIAN_POINT('',(-0.00614605578766269,-0.0225,0.0113417810883008));
#29864=CARTESIAN_POINT('',(-0.0061460557876627,-0.017,0.0113417810883008));
#29865=CARTESIAN_POINT('',(-0.00614605578767459,-0.01000000000001,0.0113417810883085));
#29866=CARTESIAN_POINT('',(-0.0052492137012165,-0.0225,0.0117837072060944));
#29867=CARTESIAN_POINT('Origin',(-0.00570191777865816,-0.02250000000001,
0.0115714361099103));
#29868=CARTESIAN_POINT('',(-0.0052492137012165,-0.017,0.0117837072060944));
#29869=CARTESIAN_POINT('',(-0.00524921370122839,-0.01000000000001,0.0117837072061021));
#29870=CARTESIAN_POINT('Origin',(-0.00570191777865816,-0.01700000000001,
0.0115714361099103));
#29871=CARTESIAN_POINT('Origin',(-0.0072568597527597,-0.01,0.0106652701104462));
#29872=CARTESIAN_POINT('',(-0.00766471363969575,-0.0225,0.0103760380117588));
#29873=CARTESIAN_POINT('',(-0.00766471363969575,-0.017,0.0103760380117588));
#29874=CARTESIAN_POINT('',(-0.00766471363970765,-0.01000000000001,0.0103760380117664));
#29875=CARTESIAN_POINT('',(-0.0068381037869931,-0.0225,0.0109384796291949));
#29876=CARTESIAN_POINT('Origin',(-0.00725685975277159,-0.02250000000001,
0.0106652701104539));
#29877=CARTESIAN_POINT('',(-0.0068381037869931,-0.017,0.0109384796291949));
#29878=CARTESIAN_POINT('',(-0.00683810378700499,-0.01000000000001,0.0109384796292026));
#29879=CARTESIAN_POINT('Origin',(-0.00725685975277159,-0.01700000000001,
0.0106652701104539));
#29880=CARTESIAN_POINT('Origin',(-0.00867055520634127,-0.01,0.00955151675985495));
#29881=CARTESIAN_POINT('',(-0.00903418655921466,-0.0225,0.00920833715788611));
#29882=CARTESIAN_POINT('',(-0.00903418655921466,-0.017,0.00920833715788611));
#29883=CARTESIAN_POINT('',(-0.00903418655922655,-0.01000000000001,0.00920833715789376));
#29884=CARTESIAN_POINT('',(-0.00829389796078363,-0.0225,0.00988034698864926));
#29885=CARTESIAN_POINT('Origin',(-0.00867055520635317,-0.02250000000001,
0.0095515167598626));
#29886=CARTESIAN_POINT('',(-0.00829389796078364,-0.017,0.00988034698864926));
#29887=CARTESIAN_POINT('',(-0.00829389796079552,-0.01000000000001,0.00988034698865692));
#29888=CARTESIAN_POINT('Origin',(-0.00867055520635317,-0.01700000000001,
0.0095515167598626));
#29889=CARTESIAN_POINT('Origin',(-0.00991548816544177,-0.01,0.0082518540002223));
#29890=CARTESIAN_POINT('',(-0.0102278193135934,-0.0225,0.00786140649556348));
#29891=CARTESIAN_POINT('',(-0.0102278193135934,-0.017,0.00786140649556348));
#29892=CARTESIAN_POINT('',(-0.0102278193136052,-0.01000000000001,0.00786140649557114));
#29893=CARTESIAN_POINT('',(-0.00958826084493661,-0.0225,0.0086299046326977));
#29894=CARTESIAN_POINT('Origin',(-0.00991548816545366,-0.02250000000001,
0.00825185400022996));
#29895=CARTESIAN_POINT('',(-0.00958826084493661,-0.017,0.0086299046326977));
#29896=CARTESIAN_POINT('',(-0.0095882608449485,-0.01000000000001,0.00862990463270536));
#29897=CARTESIAN_POINT('Origin',(-0.00991548816545366,-0.01700000000001,
0.00825185400022996));
#29898=CARTESIAN_POINT('Origin',(-0.0109674274261026,-0.01,0.0067915782888202));
#29899=CARTESIAN_POINT('',(-0.011222379199005,-0.0225,0.00636146249802205));
#29900=CARTESIAN_POINT('',(-0.011222379199005,-0.017,0.00636146249802205));
#29901=CARTESIAN_POINT('',(-0.0112223791990169,-0.01000000000001,0.00636146249802971));
#29902=CARTESIAN_POINT('',(-0.010695999138228,-0.0225,0.00721149099944164));
#29903=CARTESIAN_POINT('Origin',(-0.0109674274261145,-0.02250000000001,
0.00679157828882786));
#29904=CARTESIAN_POINT('',(-0.010695999138228,-0.017,0.00721149099944164));
#29905=CARTESIAN_POINT('',(-0.0106959991382398,-0.01000000000001,0.0072114909994493));
#29906=CARTESIAN_POINT('Origin',(-0.0109674274261145,-0.01700000000001,
0.00679157828882786));
#29907=CARTESIAN_POINT('Origin',(-0.0118058981871781,-0.01,0.005199112231332));
#29908=CARTESIAN_POINT('',(-0.0119985082385752,-0.0225,0.00473769986901296));
#29909=CARTESIAN_POINT('',(-0.0119985082385752,-0.017,0.00473769986901296));
#29910=CARTESIAN_POINT('',(-0.0119985082385871,-0.01000000000001,0.00473769986902062));
#29911=CARTESIAN_POINT('',(-0.0115955519748124,-0.0225,0.00565271389683093));
#29912=CARTESIAN_POINT('Origin',(-0.01180589818719,-0.02250000000001,0.00519911223133965));
#29913=CARTESIAN_POINT('',(-0.0115955519748124,-0.017,0.00565271389683093));
#29914=CARTESIAN_POINT('',(-0.0115955519748243,-0.01000000000001,0.00565271389683858));
#29915=CARTESIAN_POINT('Origin',(-0.01180589818719,-0.01700000000001,0.00519911223133965));
#29916=CARTESIAN_POINT('Origin',(-0.0124145805690504,-0.01,0.00350545136816342));
#29917=CARTESIAN_POINT('',(-0.0125410999633822,-0.0225,0.00302172330110727));
#29918=CARTESIAN_POINT('',(-0.0125410999633822,-0.017,0.00302172330110727));
#29919=CARTESIAN_POINT('',(-0.0125410999633941,-0.01000000000001,0.00302172330111493));
#29920=CARTESIAN_POINT('',(-0.012269410581952,-0.0225,0.00398391314808515));
#29921=CARTESIAN_POINT('Origin',(-0.0124145805690623,-0.02250000000001,
0.00350545136817107));
#29922=CARTESIAN_POINT('',(-0.012269410581952,-0.017,0.00398391314808515));
#29923=CARTESIAN_POINT('',(-0.0122694105819639,-0.01000000000001,0.00398391314809281));
#29924=CARTESIAN_POINT('Origin',(-0.0124145805690623,-0.01700000000001,
0.00350545136817107));
#29925=CARTESIAN_POINT('Origin',(-0.0127816272615221,-0.01,0.0017435608815054));
#29926=CARTESIAN_POINT('',(-0.0128395934426919,-0.0225,0.00124693232630483));
#29927=CARTESIAN_POINT('',(-0.0128395934426919,-0.017,0.00124693232630483));
#29928=CARTESIAN_POINT('',(-0.0128395934427038,-0.01000000000001,0.00124693232631249));
#29929=CARTESIAN_POINT('',(-0.0127044590683616,-0.0225,0.00223757006154593));
#29930=CARTESIAN_POINT('Origin',(-0.012781627261534,-0.02250000000001,0.00174356088151305));
#29931=CARTESIAN_POINT('',(-0.0127044590683616,-0.017,0.00223757006154593));
#29932=CARTESIAN_POINT('',(-0.0127044590683735,-0.01000000000001,0.00223757006155359));
#29933=CARTESIAN_POINT('Origin',(-0.012781627261534,-0.01700000000001,0.00174356088151305));
#29934=CARTESIAN_POINT('Origin',(-0.0128998941182339,-0.01,-5.22660344400411E-5));
#29935=CARTESIAN_POINT('',(-0.0128881788404607,-0.0225,-0.000552128767864633));
#29936=CARTESIAN_POINT('',(-0.0128881788404607,-0.017,-0.000552128767864633));
#29937=CARTESIAN_POINT('',(-0.0128881788404726,-0.01000000000001,-0.000552128767856978));
#29938=CARTESIAN_POINT('',(-0.0128922297101135,-0.0225,0.00044767521895696));
#29939=CARTESIAN_POINT('Origin',(-0.0128998941182458,-0.02250000000001,
-5.22660344323867E-5));
#29940=CARTESIAN_POINT('',(-0.0128922297101135,-0.017,0.00044767521895696));
#29941=CARTESIAN_POINT('',(-0.0128922297101254,-0.01000000000001,0.000447675218964614));
#29942=CARTESIAN_POINT('Origin',(-0.0128998941182458,-0.01700000000001,
-5.22660344323867E-5));
#29943=CARTESIAN_POINT('Origin',(-0.0127670792093463,-0.01,-0.00184707565147683));
#29944=CARTESIAN_POINT('',(-0.012685910497186,-0.0225,-0.00234044330360477));
#29945=CARTESIAN_POINT('',(-0.012685910497186,-0.017,-0.00234044330360477));
#29946=CARTESIAN_POINT('',(-0.0126859104971979,-0.01000000000001,-0.00234044330359712));
#29947=CARTESIAN_POINT('',(-0.012829067765252,-0.0225,-0.001350933112546));
#29948=CARTESIAN_POINT('Origin',(-0.0127670792093582,-0.02250000000001,
-0.00184707565146918));
#29949=CARTESIAN_POINT('',(-0.012829067765252,-0.017,-0.001350933112546));
#29950=CARTESIAN_POINT('',(-0.0128290677652638,-0.01000000000001,-0.00135093311253835));
#29951=CARTESIAN_POINT('Origin',(-0.0127670792093582,-0.01700000000001,
-0.00184707565146918));
#29952=CARTESIAN_POINT('Origin',(-0.0123857676259861,-0.01,-0.00360593404197504));
#29953=CARTESIAN_POINT('',(-0.0122367253360928,-0.0225,-0.00408320377265504));
#29954=CARTESIAN_POINT('',(-0.0122367253360928,-0.017,-0.00408320377265504));
#29955=CARTESIAN_POINT('',(-0.0122367253361005,-0.01000000000001,-0.00408320377266693));
#29956=CARTESIAN_POINT('',(-0.0125162026091882,-0.0225,-0.00312324706767692));
#29957=CARTESIAN_POINT('Origin',(-0.0123857676259938,-0.02250000000001,
-0.00360593404198693));
#29958=CARTESIAN_POINT('',(-0.0125162026091882,-0.017,-0.00312324706767692));
#29959=CARTESIAN_POINT('',(-0.0125162026091958,-0.01000000000001,-0.00312324706768881));
#29960=CARTESIAN_POINT('Origin',(-0.0123857676259938,-0.01700000000001,
-0.00360593404198693));
#29961=CARTESIAN_POINT('Origin',(-0.011763381164388,-0.01,-0.00529460702803539));
#29962=CARTESIAN_POINT('',(-0.0115493662354015,-0.0225,-0.00574648932484605));
#29963=CARTESIAN_POINT('',(-0.0115493662354015,-0.017,-0.00574648932484605));
#29964=CARTESIAN_POINT('',(-0.0115493662354091,-0.01000000000001,-0.00574648932485794));
#29965=CARTESIAN_POINT('',(-0.011959723806306,-0.0225,-0.00483477057127637));
#29966=CARTESIAN_POINT('Origin',(-0.0117633811643957,-0.02250000000001,
-0.00529460702804728));
#29967=CARTESIAN_POINT('',(-0.011959723806306,-0.017,-0.00483477057127637));
#29968=CARTESIAN_POINT('',(-0.0119597238063136,-0.01000000000001,-0.00483477057128826));
#29969=CARTESIAN_POINT('Origin',(-0.0117633811643957,-0.01700000000001,
-0.00529460702804728));
#29970=CARTESIAN_POINT('Origin',(-0.0109120338690729,-0.01,-0.00688022651082125));
#29971=CARTESIAN_POINT('',(-0.0106372118581474,-0.0225,-0.00729792599886364));
#29972=CARTESIAN_POINT('',(-0.0106372118581474,-0.017,-0.00729792599886364));
#29973=CARTESIAN_POINT('',(-0.010637211858155,-0.01000000000001,-0.00729792599887552));
#29974=CARTESIAN_POINT('',(-0.0111704625835182,-0.0225,-0.00645219076517593));
#29975=CARTESIAN_POINT('Origin',(-0.0109120338690805,-0.02250000000001,
-0.00688022651083314));
#29976=CARTESIAN_POINT('',(-0.0111704625835182,-0.017,-0.00645219076517593));
#29977=CARTESIAN_POINT('',(-0.0111704625835258,-0.01000000000001,-0.00645219076518782));
#29978=CARTESIAN_POINT('Origin',(-0.0109120338690805,-0.01700000000001,
-0.00688022651083314));
#29979=CARTESIAN_POINT('Origin',(-0.0098482962467508,-0.01,-0.00833193021071565));
#29980=CARTESIAN_POINT('',(-0.0095180162517236,-0.0225,-0.00870731684458113));
#29981=CARTESIAN_POINT('',(-0.0095180162517236,-0.017,-0.00870731684458113));
#29982=CARTESIAN_POINT('',(-0.00951801625173126,-0.01000000000001,-0.00870731684459302));
#29983=CARTESIAN_POINT('',(-0.0101637810127551,-0.0225,-0.00794402640508956));
#29984=CARTESIAN_POINT('Origin',(-0.00984829624675845,-0.02250000000001,
-0.00833193021072754));
#29985=CARTESIAN_POINT('',(-0.0101637810127551,-0.017,-0.00794402640508956));
#29986=CARTESIAN_POINT('',(-0.0101637810127627,-0.01000000000001,-0.00794402640510145));
#29987=CARTESIAN_POINT('Origin',(-0.00984829624675845,-0.01700000000001,
-0.00833193021072754));
#29988=CARTESIAN_POINT('Origin',(-0.00859287274025656,-0.01,-0.00962146236648858));
#29989=CARTESIAN_POINT('',(-0.00821356328554307,-0.0225,-0.00994722967234497));
#29990=CARTESIAN_POINT('',(-0.00821356328554307,-0.017,-0.00994722967234497));
#29991=CARTESIAN_POINT('',(-0.00821356328555072,-0.01000000000001,-0.00994722967235687));
#29992=CARTESIAN_POINT('',(-0.00895927300570829,-0.0225,-0.00928124060722424));
#29993=CARTESIAN_POINT('Origin',(-0.00859287274026421,-0.02250000000001,
-0.00962146236650047));
#29994=CARTESIAN_POINT('',(-0.00895927300570829,-0.017,-0.00928124060722424));
#29995=CARTESIAN_POINT('',(-0.00895927300571595,-0.01000000000001,-0.00928124060723613));
#29996=CARTESIAN_POINT('Origin',(-0.00859287274026421,-0.01700000000001,
-0.00962146236650047));
#29997=CARTESIAN_POINT('Origin',(-0.00717019874012118,-0.01,-0.0107237237015491));
#29998=CARTESIAN_POINT('',(-0.00674924265279915,-0.0225,-0.0109935309893427));
#29999=CARTESIAN_POINT('',(-0.00674924265279915,-0.017,-0.0109935309893427));
#30000=CARTESIAN_POINT('',(-0.00674924265280681,-0.01000000000001,-0.0109935309893545));
#30001=CARTESIAN_POINT('',(-0.00758038294062733,-0.0225,-0.010437806018194));
#30002=CARTESIAN_POINT('Origin',(-0.00717019874012884,-0.02250000000001,
-0.010723723701561));
#30003=CARTESIAN_POINT('',(-0.00758038294062733,-0.017,-0.010437806018194));
#30004=CARTESIAN_POINT('',(-0.00758038294063499,-0.01000000000001,-0.0104378060182059));
#30005=CARTESIAN_POINT('Origin',(-0.00717019874012884,-0.01700000000001,
-0.010723723701561));
#30006=CARTESIAN_POINT('Origin',(-0.00560796497748951,-0.01,-0.0116172599528138));
#30007=CARTESIAN_POINT('',(-0.00515355568896825,-0.0225,-0.011825855730589));
#30008=CARTESIAN_POINT('',(-0.00515355568896825,-0.017,-0.011825855730589));
#30009=CARTESIAN_POINT('',(-0.0051535556889759,-0.01000000000001,-0.0118258557306009));
#30010=CARTESIAN_POINT('',(-0.00605394934416489,-0.0225,-0.011391211407848));
#30011=CARTESIAN_POINT('Origin',(-0.00560796497749716,-0.02250000000001,
-0.0116172599528257));
#30012=CARTESIAN_POINT('',(-0.00605394934416489,-0.017,-0.011391211407848));
#30013=CARTESIAN_POINT('',(-0.00605394934417254,-0.01000000000001,-0.0113912114078599));
#30014=CARTESIAN_POINT('Origin',(-0.00560796497749716,-0.01700000000001,
-0.0116172599528257));
#30015=CARTESIAN_POINT('Origin',(-0.00393657855553661,-0.01,-0.0122846794535344));
#30016=CARTESIAN_POINT('',(-0.00345756062573429,-0.0225,-0.0124280036417509));
#30017=CARTESIAN_POINT('',(-0.00345756062573429,-0.017,-0.0124280036417509));
#30018=CARTESIAN_POINT('',(-0.00345756062574195,-0.01000000000001,-0.0124280036417628));
#30019=CARTESIAN_POINT('',(-0.00440968250998358,-0.0225,-0.0121228998247591));
#30020=CARTESIAN_POINT('Origin',(-0.00393657855554426,-0.02250000000001,
-0.0122846794535463));
#30021=CARTESIAN_POINT('',(-0.00440968250998358,-0.017,-0.0121228998247591));
#30022=CARTESIAN_POINT('',(-0.00440968250999122,-0.01000000000001,-0.012122899824771));
#30023=CARTESIAN_POINT('Origin',(-0.00393657855554426,-0.01700000000001,
-0.0122846794535463));
#30024=CARTESIAN_POINT('Origin',(-0.00218857110979193,-0.01,-0.0127129916423077));
#30025=CARTESIAN_POINT('',(-0.00169426807783735,-0.0225,-0.0127882545986707));
#30026=CARTESIAN_POINT('',(-0.00169426807783735,-0.017,-0.0127882545986707));
#30027=CARTESIAN_POINT('',(-0.00169426807784501,-0.01000000000001,-0.0127882545986826));
#30028=CARTESIAN_POINT('',(-0.00267958622168495,-0.0225,-0.0126186297861756));
#30029=CARTESIAN_POINT('Origin',(-0.00218857110979959,-0.02250000000001,
-0.0127129916423196));
#30030=CARTESIAN_POINT('',(-0.00267958622168495,-0.017,-0.0126186297861756));
#30031=CARTESIAN_POINT('',(-0.0026795862216926,-0.01000000000001,-0.0126186297861875));
#30032=CARTESIAN_POINT('Origin',(-0.00218857110979959,-0.01700000000001,
-0.0127129916423196));
#30033=CARTESIAN_POINT('Origin',(-0.000397965616857901,-0.01,-0.0128938599095771));
#30034=CARTESIAN_POINT('',(0.000102001470993324,-0.0225,-0.0128995967262514));
#30035=CARTESIAN_POINT('',(0.000102001470993324,-0.017,-0.0128995967262514));
#30036=CARTESIAN_POINT('',(0.000102001470985668,-0.01000000000001,-0.0128995967262633));
#30037=CARTESIAN_POINT('',(-0.000897334835565392,-0.0225,-0.0128687524722826));
#30038=CARTESIAN_POINT('Origin',(-0.000397965616865555,-0.02250000000001,
-0.012893859909589));
#30039=CARTESIAN_POINT('',(-0.000897334835565393,-0.017,-0.0128687524722826));
#30040=CARTESIAN_POINT('',(-0.000897334835573037,-0.01000000000001,-0.0128687524722945));
#30041=CARTESIAN_POINT('Origin',(-0.000397965616865556,-0.01700000000001,
-0.012893859909589));
#30042=CARTESIAN_POINT('Origin',(0.00140038582412907,-0.01,-0.0128237638602548));
#30043=CARTESIAN_POINT('',(0.00189628567721606,-0.0225,-0.0127598628766294));
#30044=CARTESIAN_POINT('',(0.00189628567721606,-0.017,-0.0127598628766294));
#30045=CARTESIAN_POINT('',(0.0018962856772084,-0.01000000000001,-0.0127598628766413));
#30046=CARTESIAN_POINT('',(0.000902382152425214,-0.0225,-0.0128683995295057));
#30047=CARTESIAN_POINT('Origin',(0.00140038582412142,-0.02250000000001,
-0.0128237638602667));
#30048=CARTESIAN_POINT('',(0.000902382152425214,-0.017,-0.0128683995295057));
#30049=CARTESIAN_POINT('',(0.000902382152417559,-0.01000000000001,-0.0128683995295176));
#30050=CARTESIAN_POINT('Origin',(0.00140038582412142,-0.01700000000001,
-0.0128237638602667));
#30051=CARTESIAN_POINT('Origin',(0.00317148034796465,-0.01,-0.0125040678342079));
#30052=CARTESIAN_POINT('',(0.0036536608397248,-0.0225,-0.0123717728102428));
#30053=CARTESIAN_POINT('',(0.0036536608397248,-0.017,-0.0123717728102428));
#30054=CARTESIAN_POINT('',(0.00365366083973669,-0.01000000000001,-0.0123717728102504));
#30055=CARTESIAN_POINT('',(0.00268453529826336,-0.0225,-0.0126175778274746));
#30056=CARTESIAN_POINT('Origin',(0.00317148034797655,-0.02250000000001,
-0.0125040678342156));
#30057=CARTESIAN_POINT('',(0.00268453529826336,-0.017,-0.0126175778274746));
#30058=CARTESIAN_POINT('',(0.0026845352982557,-0.01000000000001,-0.0126175778274865));
#30059=CARTESIAN_POINT('Origin',(0.00317148034797655,-0.01700000000001,
-0.0125040678342156));
#30060=CARTESIAN_POINT('Origin',(0.00488084561433254,-0.01,-0.0119409943509345));
#30061=CARTESIAN_POINT('',(0.00533992164996588,-0.0225,-0.0117428802587877));
#30062=CARTESIAN_POINT('',(0.00533992164996587,-0.017,-0.0117428802587877));
#30063=CARTESIAN_POINT('',(0.00533992164997777,-0.01000000000001,-0.0117428802587953));
#30064=CARTESIAN_POINT('',(0.00441443701813444,-0.0225,-0.0121211693253137));
#30065=CARTESIAN_POINT('Origin',(0.00488084561434443,-0.02250000000001,
-0.0119409943509422));
#30066=CARTESIAN_POINT('',(0.00441443701813444,-0.017,-0.0121211693253137));
#30067=CARTESIAN_POINT('',(0.00441443701814632,-0.01000000000001,-0.0121211693253213));
#30068=CARTESIAN_POINT('Origin',(0.00488084561434443,-0.01700000000001,
-0.0119409943509422));
#30069=CARTESIAN_POINT('Origin',(0.00649521077269703,-0.01,-0.0111455029953));
#30070=CARTESIAN_POINT('',(0.00692224695936122,-0.0225,-0.0108854259004236));
#30071=CARTESIAN_POINT('',(0.00692224695936122,-0.017,-0.0108854259004236));
#30072=CARTESIAN_POINT('',(0.00692224695937311,-0.01000000000001,-0.0108854259004312));
#30073=CARTESIAN_POINT('',(0.00605841674279519,-0.0225,-0.0113888360498612));
#30074=CARTESIAN_POINT('Origin',(0.00649521077270892,-0.02250000000001,
-0.0111455029953076));
#30075=CARTESIAN_POINT('',(0.00605841674279519,-0.017,-0.0113888360498612));
#30076=CARTESIAN_POINT('',(0.00605841674280708,-0.01000000000001,-0.0113888360498688));
#30077=CARTESIAN_POINT('Origin',(0.00649521077270892,-0.01700000000001,
-0.0111455029953076));
#30078=CARTESIAN_POINT('Origin',(0.00798315404156373,-0.01,-0.0101330771016836));
#30079=CARTESIAN_POINT('',(0.00836983860563182,-0.0225,-0.0098160991088963));
#30080=CARTESIAN_POINT('',(0.00836983860563182,-0.017,-0.0098160991088963));
#30081=CARTESIAN_POINT('',(0.00836983860564371,-0.01000000000001,-0.00981609910890396));
#30082=CARTESIAN_POINT('',(0.00758447627690437,-0.0225,-0.0104348320353073));
#30083=CARTESIAN_POINT('Origin',(0.00798315404157562,-0.02250000000001,
-0.0101330771016913));
#30084=CARTESIAN_POINT('',(0.00758447627690437,-0.017,-0.0104348320353073));
#30085=CARTESIAN_POINT('',(0.00758447627691626,-0.01000000000001,-0.0104348320353149));
#30086=CARTESIAN_POINT('Origin',(0.00798315404157562,-0.01700000000001,
-0.0101330771016913));
#30087=CARTESIAN_POINT('Origin',(0.00931571429771449,-0.01,-0.00892342238848729));
#30088=CARTESIAN_POINT('',(0.00965452086399409,-0.0225,-0.00855571311386156));
#30089=CARTESIAN_POINT('',(0.00965452086399409,-0.017,-0.00855571311386156));
#30090=CARTESIAN_POINT('',(0.00965452086400598,-0.01000000000001,-0.00855571311386922));
#30091=CARTESIAN_POINT('',(0.00896291260749749,-0.0225,-0.00927772588463158));
#30092=CARTESIAN_POINT('Origin',(0.00931571429772638,-0.02250000000001,
-0.00892342238849495));
#30093=CARTESIAN_POINT('',(0.00896291260749749,-0.017,-0.00927772588463158));
#30094=CARTESIAN_POINT('',(0.00896291260750938,-0.01000000000001,-0.00927772588463924));
#30095=CARTESIAN_POINT('Origin',(0.00931571429772638,-0.01700000000001,
-0.00892342238849495));
#30096=CARTESIAN_POINT('Origin',(0.0104669547715282,-0.01,-0.00754008340874168));
#30097=CARTESIAN_POINT('',(0.0107512888555934,-0.0225,-0.00712879989504486));
#30098=CARTESIAN_POINT('',(0.0107512888555934,-0.017,-0.00712879989504486));
#30099=CARTESIAN_POINT('',(0.0107512888556053,-0.01000000000001,-0.00712879989505252));
#30100=CARTESIAN_POINT('',(0.0101668960393476,-0.0225,-0.00794003935286826));
#30101=CARTESIAN_POINT('Origin',(0.0104669547715401,-0.02250000000001,-0.00754008340874933));
#30102=CARTESIAN_POINT('',(0.0101668960393476,-0.017,-0.00794003935286826));
#30103=CARTESIAN_POINT('',(0.0101668960393595,-0.01000000000001,-0.00794003935287591));
#30104=CARTESIAN_POINT('Origin',(0.0104669547715401,-0.01700000000001,-0.00754008340874933));
#30105=CARTESIAN_POINT('Origin',(0.0114144678766987,-0.01,-0.00600998528216265));
#30106=CARTESIAN_POINT('',(0.0116387952390284,-0.0225,-0.00556313269516086));
#30107=CARTESIAN_POINT('',(0.0116387952390284,-0.017,-0.00556313269516086));
#30108=CARTESIAN_POINT('',(0.0116387952390403,-0.01000000000001,-0.00556313269516851));
#30109=CARTESIAN_POINT('',(0.0111729924044647,-0.0225,-0.00644780898676229));
#30110=CARTESIAN_POINT('Origin',(0.0114144678767106,-0.02250000000001,-0.0060099852821703));
#30111=CARTESIAN_POINT('',(0.0111729924044647,-0.017,-0.00644780898676229));
#30112=CARTESIAN_POINT('',(0.0111729924044766,-0.01000000000001,-0.00644780898676994));
#30113=CARTESIAN_POINT('Origin',(0.0114144678767106,-0.01700000000001,-0.0060099852821703));
#30114=CARTESIAN_POINT('Origin',(0.0121398113484141,-0.01,-0.00436290962832323));
#30115=CARTESIAN_POINT('',(0.0122997657120691,-0.0225,-0.00388918544533519));
#30116=CARTESIAN_POINT('',(0.0122997657120691,-0.017,-0.00388918544533519));
#30117=CARTESIAN_POINT('',(0.012299765712081,-0.01000000000001,-0.00388918544534284));
#30118=CARTESIAN_POINT('',(0.0119616191815194,-0.0225,-0.004830079353003));
#30119=CARTESIAN_POINT('Origin',(0.012139811348426,-0.02250000000001,-0.00436290962833088));
#30120=CARTESIAN_POINT('',(0.0119616191815194,-0.017,-0.004830079353003));
#30121=CARTESIAN_POINT('',(0.0119616191815313,-0.01000000000001,-0.00483007935301066));
#30122=CARTESIAN_POINT('Origin',(0.012139811348426,-0.01700000000001,-0.00436290962833088));
#30123=CARTESIAN_POINT('Origin',(0.0126288672010633,-0.01,-0.00263091490130466));
#30124=CARTESIAN_POINT('',(0.0127213352363006,-0.0225,-0.00213953962469893));
#30125=CARTESIAN_POINT('',(0.0127213352363006,-0.017,-0.00213953962469893));
#30126=CARTESIAN_POINT('',(0.0127213352363125,-0.01000000000001,-0.00213953962470658));
#30127=CARTESIAN_POINT('',(0.012517426647346,-0.0225,-0.00311833771877137));
#30128=CARTESIAN_POINT('Origin',(0.0126288672010752,-0.02250000000001,-0.00263091490131231));
#30129=CARTESIAN_POINT('',(0.012517426647346,-0.017,-0.00311833771877137));
#30130=CARTESIAN_POINT('',(0.0125174266473579,-0.01000000000001,-0.00311833771877902));
#30131=CARTESIAN_POINT('Origin',(0.0126288672010752,-0.01700000000001,-0.00263091490131231));
#30132=CARTESIAN_POINT('Origin',(0.0128721165187673,-0.01,-0.000847712408353549));
#30133=CARTESIAN_POINT('',(0.0128952984404617,-0.0225,-0.000348250098958184));
#30134=CARTESIAN_POINT('',(0.0128952984404617,-0.017,-0.000348250098958184));
#30135=CARTESIAN_POINT('',(0.0128952984404736,-0.01000000000001,-0.000348250098965837));
#30136=CARTESIAN_POINT('',(0.0128295966418437,-0.0225,-0.00134590118790042));
#30137=CARTESIAN_POINT('Origin',(0.0128721165187792,-0.02250000000001,-0.000847712408361203));
#30138=CARTESIAN_POINT('',(0.0128295966418437,-0.017,-0.00134590118790042));
#30139=CARTESIAN_POINT('',(0.0128295966418555,-0.01000000000001,-0.00134590118790808));
#30140=CARTESIAN_POINT('Origin',(0.0128721165187792,-0.01700000000001,-0.000847712408361203));
#30141=CARTESIAN_POINT('Origin',(0.0128648247302491,-0.01,0.000951989842367618));
#30142=CARTESIAN_POINT('',(0.0128182693286638,-0.0225,0.00144981771883018));
#30143=CARTESIAN_POINT('',(0.0128182693286638,-0.017,0.00144981771883018));
#30144=CARTESIAN_POINT('',(0.0128182693286757,-0.01000000000001,0.00144981771882252));
#30145=CARTESIAN_POINT('',(0.0128920531311578,-0.0225,0.000452731778653103));
#30146=CARTESIAN_POINT('Origin',(0.012864824730261,-0.02250000000001,0.000951989842359964));
#30147=CARTESIAN_POINT('',(0.0128920531311578,-0.017,0.000452731778653103));
#30148=CARTESIAN_POINT('',(0.0128920531311697,-0.01000000000001,0.000452731778645449));
#30149=CARTESIAN_POINT('Origin',(0.012864824730261,-0.01700000000001,0.000951989842359964));
#30150=CARTESIAN_POINT('Origin',(-4.42567805516485E-17,-0.017,1.23897393496637E-32));
#30151=CARTESIAN_POINT('',(0.0124917471849488,-0.017,0.00321966648386474));
#30152=CARTESIAN_POINT('Origin',(-4.42567805516478E-17,-0.01700000000001,
1.23897393496654E-32));
#30153=CARTESIAN_POINT('',(0.0127035804707671,-0.017,0.00224255283610991));
#30154=CARTESIAN_POINT('Origin',(0.0126071337618875,-0.01700000000001,0.00273316269368159));
#30155=CARTESIAN_POINT('Origin',(-4.42567805516478E-17,-0.01700000000001,
1.23897393496654E-32));
#30156=CARTESIAN_POINT('Origin',(-4.42567805516478E-17,-0.01700000000001,
1.23897393496654E-32));
#30157=CARTESIAN_POINT('Origin',(-4.42567805516478E-17,-0.01700000000001,
1.23897393496654E-32));
#30158=CARTESIAN_POINT('Origin',(-4.42567805516478E-17,-0.01700000000001,
1.23897393496654E-32));
#30159=CARTESIAN_POINT('Origin',(-4.42567805516478E-17,-0.01700000000001,
1.23897393496654E-32));
#30160=CARTESIAN_POINT('Origin',(-4.42567805516478E-17,-0.01700000000001,
1.23897393496654E-32));
#30161=CARTESIAN_POINT('Origin',(-4.42567805516478E-17,-0.01700000000001,
1.23897393496654E-32));
#30162=CARTESIAN_POINT('Origin',(-4.42567805516478E-17,-0.01700000000001,
1.23897393496654E-32));
#30163=CARTESIAN_POINT('Origin',(-4.42567805516478E-17,-0.01700000000001,
1.23897393496654E-32));
#30164=CARTESIAN_POINT('Origin',(-4.42567805516478E-17,-0.01700000000001,
1.23897393496654E-32));
#30165=CARTESIAN_POINT('Origin',(-4.42567805516478E-17,-0.01700000000001,
1.23897393496654E-32));
#30166=CARTESIAN_POINT('Origin',(-4.42567805516478E-17,-0.01700000000001,
1.23897393496654E-32));
#30167=CARTESIAN_POINT('Origin',(-4.42567805516478E-17,-0.01700000000001,
1.23897393496654E-32));
#30168=CARTESIAN_POINT('Origin',(-4.42567805516478E-17,-0.01700000000001,
1.23897393496654E-32));
#30169=CARTESIAN_POINT('Origin',(-4.42567805516478E-17,-0.01700000000001,
1.23897393496654E-32));
#30170=CARTESIAN_POINT('Origin',(-4.42567805516478E-17,-0.01700000000001,
1.23897393496654E-32));
#30171=CARTESIAN_POINT('Origin',(-4.42567805516478E-17,-0.01700000000001,
1.23897393496654E-32));
#30172=CARTESIAN_POINT('Origin',(-4.42567805516478E-17,-0.01700000000001,
1.23897393496654E-32));
#30173=CARTESIAN_POINT('Origin',(-4.42567805516478E-17,-0.01700000000001,
1.23897393496654E-32));
#30174=CARTESIAN_POINT('Origin',(-4.42567805516478E-17,-0.01700000000001,
1.23897393496654E-32));
#30175=CARTESIAN_POINT('Origin',(-4.42567805516478E-17,-0.01700000000001,
1.23897393496654E-32));
#30176=CARTESIAN_POINT('Origin',(-4.42567805516478E-17,-0.01700000000001,
1.23897393496654E-32));
#30177=CARTESIAN_POINT('Origin',(-4.42567805516478E-17,-0.01700000000001,
1.23897393496654E-32));
#30178=CARTESIAN_POINT('Origin',(-4.42567805516478E-17,-0.01700000000001,
1.23897393496654E-32));
#30179=CARTESIAN_POINT('Origin',(-4.42567805516478E-17,-0.01700000000001,
1.23897393496654E-32));
#30180=CARTESIAN_POINT('Origin',(-4.42567805516478E-17,-0.01700000000001,
1.23897393496654E-32));
#30181=CARTESIAN_POINT('Origin',(-4.42567805516478E-17,-0.01700000000001,
1.23897393496654E-32));
#30182=CARTESIAN_POINT('Origin',(-4.42567805516478E-17,-0.01700000000001,
1.23897393496654E-32));
#30183=CARTESIAN_POINT('Origin',(-4.42567805516478E-17,-0.01700000000001,
1.23897393496654E-32));
#30184=CARTESIAN_POINT('Origin',(-4.42567805516478E-17,-0.01700000000001,
1.23897393496654E-32));
#30185=CARTESIAN_POINT('Origin',(-4.42567805516478E-17,-0.01700000000001,
1.23897393496654E-32));
#30186=CARTESIAN_POINT('Origin',(-4.42567805516478E-17,-0.01700000000001,
1.23897393496654E-32));
#30187=CARTESIAN_POINT('Origin',(-4.42567805516478E-17,-0.01700000000001,
1.23897393496654E-32));
#30188=CARTESIAN_POINT('Origin',(-4.42567805516478E-17,-0.01700000000001,
1.23897393496654E-32));
#30189=CARTESIAN_POINT('Origin',(-4.42567805516478E-17,-0.01700000000001,
1.23897393496654E-32));
#30190=CARTESIAN_POINT('Origin',(-4.42567805516478E-17,-0.01700000000001,
1.23897393496654E-32));
#30191=CARTESIAN_POINT('Origin',(-4.42567805516478E-17,-0.01700000000001,
1.23897393496654E-32));
#30192=CARTESIAN_POINT('Origin',(-4.42567805516478E-17,-0.01700000000001,
1.23897393496654E-32));
#30193=CARTESIAN_POINT('Origin',(-4.42567805516478E-17,-0.01700000000001,
1.23897393496654E-32));
#30194=CARTESIAN_POINT('Origin',(-4.42567805516478E-17,-0.01700000000001,
1.23897393496654E-32));
#30195=CARTESIAN_POINT('Origin',(-4.42567805516478E-17,-0.01700000000001,
1.23897393496654E-32));
#30196=CARTESIAN_POINT('Origin',(-4.42567805516478E-17,-0.01700000000001,
1.23897393496654E-32));
#30197=CARTESIAN_POINT('Origin',(-4.42567805516478E-17,-0.01700000000001,
1.23897393496654E-32));
#30198=CARTESIAN_POINT('Origin',(-4.42567805516478E-17,-0.01700000000001,
1.23897393496654E-32));
#30199=CARTESIAN_POINT('',(-0.000529682692573584,-0.01700000000001,0.0024432429771081));
#30200=CARTESIAN_POINT('Origin',(-4.42567805516478E-17,-0.01700000000001,
1.23897393496654E-32));
#30201=CARTESIAN_POINT('Origin',(-4.38905912375397E-17,-0.0225,1.33303635345025E-32));
#30202=CARTESIAN_POINT('',(0.0124917471849488,-0.0225,0.00321966648386474));
#30203=CARTESIAN_POINT('Origin',(-4.38905912375391E-17,-0.02250000000001,
1.33303635345042E-32));
#30204=CARTESIAN_POINT('',(0.0124917471849565,-0.01000000000001,0.00321966648387663));
#30205=CARTESIAN_POINT('Origin',(-4.38905912375397E-17,-0.0225,1.33303635345025E-32));
#30206=CARTESIAN_POINT('',(0.0127035804707671,-0.0225,0.00224255283610991));
#30207=CARTESIAN_POINT('',(0.012703580470779,-0.01000000000001,0.00224255283610226));
#30208=CARTESIAN_POINT('Origin',(-4.38905912375391E-17,-0.02250000000001,
1.33303635345042E-32));
#30209=CARTESIAN_POINT('Origin',(-4.38905912375397E-17,-0.0225,1.33303635345025E-32));
#30210=CARTESIAN_POINT('Origin',(-4.38905912375391E-17,-0.02250000000001,
1.33303635345042E-32));
#30211=CARTESIAN_POINT('Origin',(-4.38905912375397E-17,-0.0225,1.33303635345025E-32));
#30212=CARTESIAN_POINT('Origin',(-4.38905912375391E-17,-0.02250000000001,
1.33303635345042E-32));
#30213=CARTESIAN_POINT('Origin',(-4.38905912375397E-17,-0.0225,1.33303635345025E-32));
#30214=CARTESIAN_POINT('Origin',(-4.38905912375391E-17,-0.02250000000001,
1.33303635345042E-32));
#30215=CARTESIAN_POINT('Origin',(-4.38905912375397E-17,-0.0225,1.33303635345025E-32));
#30216=CARTESIAN_POINT('Origin',(-4.38905912375391E-17,-0.02250000000001,
1.33303635345042E-32));
#30217=CARTESIAN_POINT('Origin',(-4.38905912375397E-17,-0.0225,1.33303635345025E-32));
#30218=CARTESIAN_POINT('Origin',(-4.38905912375391E-17,-0.02250000000001,
1.33303635345042E-32));
#30219=CARTESIAN_POINT('Origin',(-4.38905912375397E-17,-0.0225,1.33303635345025E-32));
#30220=CARTESIAN_POINT('Origin',(-4.38905912375391E-17,-0.02250000000001,
1.33303635345042E-32));
#30221=CARTESIAN_POINT('Origin',(-4.38905912375397E-17,-0.0225,1.33303635345025E-32));
#30222=CARTESIAN_POINT('Origin',(-4.38905912375391E-17,-0.02250000000001,
1.33303635345042E-32));
#30223=CARTESIAN_POINT('Origin',(-4.38905912375397E-17,-0.0225,1.33303635345025E-32));
#30224=CARTESIAN_POINT('Origin',(-4.38905912375391E-17,-0.02250000000001,
1.33303635345042E-32));
#30225=CARTESIAN_POINT('Origin',(-4.38905912375397E-17,-0.0225,1.33303635345025E-32));
#30226=CARTESIAN_POINT('Origin',(-4.38905912375391E-17,-0.02250000000001,
1.33303635345042E-32));
#30227=CARTESIAN_POINT('Origin',(-4.38905912375397E-17,-0.0225,1.33303635345025E-32));
#30228=CARTESIAN_POINT('Origin',(-4.38905912375391E-17,-0.02250000000001,
1.33303635345042E-32));
#30229=CARTESIAN_POINT('Origin',(-4.38905912375397E-17,-0.0225,1.33303635345025E-32));
#30230=CARTESIAN_POINT('Origin',(-4.38905912375391E-17,-0.02250000000001,
1.33303635345042E-32));
#30231=CARTESIAN_POINT('Origin',(-4.38905912375397E-17,-0.0225,1.33303635345025E-32));
#30232=CARTESIAN_POINT('Origin',(-4.38905912375391E-17,-0.02250000000001,
1.33303635345042E-32));
#30233=CARTESIAN_POINT('Origin',(-4.38905912375397E-17,-0.0225,1.33303635345025E-32));
#30234=CARTESIAN_POINT('Origin',(-4.38905912375391E-17,-0.02250000000001,
1.33303635345042E-32));
#30235=CARTESIAN_POINT('Origin',(-4.38905912375397E-17,-0.0225,1.33303635345025E-32));
#30236=CARTESIAN_POINT('Origin',(-4.38905912375391E-17,-0.02250000000001,
1.33303635345042E-32));
#30237=CARTESIAN_POINT('Origin',(-4.38905912375397E-17,-0.0225,1.33303635345025E-32));
#30238=CARTESIAN_POINT('Origin',(-4.38905912375391E-17,-0.02250000000001,
1.33303635345042E-32));
#30239=CARTESIAN_POINT('Origin',(-4.38905912375397E-17,-0.0225,1.33303635345025E-32));
#30240=CARTESIAN_POINT('Origin',(-4.38905912375391E-17,-0.02250000000001,
1.33303635345042E-32));
#30241=CARTESIAN_POINT('Origin',(-4.38905912375397E-17,-0.0225,1.33303635345025E-32));
#30242=CARTESIAN_POINT('Origin',(-4.38905912375391E-17,-0.02250000000001,
1.33303635345042E-32));
#30243=CARTESIAN_POINT('Origin',(-4.38905912375397E-17,-0.0225,1.33303635345025E-32));
#30244=CARTESIAN_POINT('Origin',(-4.38905912375391E-17,-0.02250000000001,
1.33303635345042E-32));
#30245=CARTESIAN_POINT('Origin',(-4.38905912375397E-17,-0.0225,1.33303635345025E-32));
#30246=CARTESIAN_POINT('Origin',(-4.38905912375391E-17,-0.02250000000001,
1.33303635345042E-32));
#30247=CARTESIAN_POINT('Origin',(-4.38905912375397E-17,-0.0225,1.33303635345025E-32));
#30248=CARTESIAN_POINT('Origin',(-4.38905912375391E-17,-0.02250000000001,
1.33303635345042E-32));
#30249=CARTESIAN_POINT('Origin',(-4.38905912375397E-17,-0.0225,1.33303635345025E-32));
#30250=CARTESIAN_POINT('Origin',(-4.38905912375391E-17,-0.02250000000001,
1.33303635345042E-32));
#30251=CARTESIAN_POINT('Origin',(-4.38905912375397E-17,-0.0225,1.33303635345025E-32));
#30252=CARTESIAN_POINT('Origin',(-4.38905912375391E-17,-0.02250000000001,
1.33303635345042E-32));
#30253=CARTESIAN_POINT('Origin',(-4.38905912375397E-17,-0.0225,1.33303635345025E-32));
#30254=CARTESIAN_POINT('Origin',(-4.38905912375391E-17,-0.02250000000001,
1.33303635345042E-32));
#30255=CARTESIAN_POINT('Origin',(-4.38905912375397E-17,-0.0225,1.33303635345025E-32));
#30256=CARTESIAN_POINT('Origin',(-4.38905912375391E-17,-0.02250000000001,
1.33303635345042E-32));
#30257=CARTESIAN_POINT('Origin',(-4.38905912375397E-17,-0.0225,1.33303635345025E-32));
#30258=CARTESIAN_POINT('Origin',(-4.38905912375391E-17,-0.02250000000001,
1.33303635345042E-32));
#30259=CARTESIAN_POINT('Origin',(-4.38905912375397E-17,-0.0225,1.33303635345025E-32));
#30260=CARTESIAN_POINT('Origin',(-4.38905912375391E-17,-0.02250000000001,
1.33303635345042E-32));
#30261=CARTESIAN_POINT('Origin',(-4.38905912375397E-17,-0.0225,1.33303635345025E-32));
#30262=CARTESIAN_POINT('Origin',(-4.38905912375391E-17,-0.02250000000001,
1.33303635345042E-32));
#30263=CARTESIAN_POINT('Origin',(-4.38905912375397E-17,-0.0225,1.33303635345025E-32));
#30264=CARTESIAN_POINT('Origin',(-4.38905912375391E-17,-0.02250000000001,
1.33303635345042E-32));
#30265=CARTESIAN_POINT('Origin',(-4.38905912375397E-17,-0.0225,1.33303635345025E-32));
#30266=CARTESIAN_POINT('Origin',(-4.38905912375391E-17,-0.02250000000001,
1.33303635345042E-32));
#30267=CARTESIAN_POINT('Origin',(-4.38905912375397E-17,-0.0225,1.33303635345025E-32));
#30268=CARTESIAN_POINT('Origin',(-4.38905912375391E-17,-0.02250000000001,
1.33303635345042E-32));
#30269=CARTESIAN_POINT('Origin',(-4.38905912375397E-17,-0.0225,1.33303635345025E-32));
#30270=CARTESIAN_POINT('Origin',(-4.38905912375391E-17,-0.02250000000001,
1.33303635345042E-32));
#30271=CARTESIAN_POINT('Origin',(-4.38905912375397E-17,-0.0225,1.33303635345025E-32));
#30272=CARTESIAN_POINT('Origin',(-4.38905912375391E-17,-0.02250000000001,
1.33303635345042E-32));
#30273=CARTESIAN_POINT('Origin',(-4.38905912375397E-17,-0.0225,1.33303635345025E-32));
#30274=CARTESIAN_POINT('Origin',(-4.38905912375391E-17,-0.02250000000001,
1.33303635345042E-32));
#30275=CARTESIAN_POINT('Origin',(-4.38905912375397E-17,-0.0225,1.33303635345025E-32));
#30276=CARTESIAN_POINT('Origin',(-4.38905912375391E-17,-0.02250000000001,
1.33303635345042E-32));
#30277=CARTESIAN_POINT('Origin',(-4.38905912375397E-17,-0.0225,1.33303635345025E-32));
#30278=CARTESIAN_POINT('Origin',(-4.38905912375391E-17,-0.02250000000001,
1.33303635345042E-32));
#30279=CARTESIAN_POINT('Origin',(-4.38905912375397E-17,-0.0225,1.33303635345025E-32));
#30280=CARTESIAN_POINT('Origin',(-4.38905912375391E-17,-0.02250000000001,
1.33303635345042E-32));
#30281=CARTESIAN_POINT('Origin',(-4.38905912375397E-17,-0.0225,1.33303635345025E-32));
#30282=CARTESIAN_POINT('Origin',(-4.38905912375391E-17,-0.02250000000001,
1.33303635345042E-32));
#30283=CARTESIAN_POINT('Origin',(-4.38905912375397E-17,-0.0225,1.33303635345025E-32));
#30284=CARTESIAN_POINT('Origin',(-4.38905912375391E-17,-0.02250000000001,
1.33303635345042E-32));
#30285=CARTESIAN_POINT('Origin',(-4.38905912375397E-17,-0.0225,1.33303635345025E-32));
#30286=CARTESIAN_POINT('Origin',(-4.38905912375391E-17,-0.02250000000001,
1.33303635345042E-32));
#30287=CARTESIAN_POINT('Origin',(-4.38905912375397E-17,-0.0225,1.33303635345025E-32));
#30288=CARTESIAN_POINT('Origin',(-4.38905912375391E-17,-0.02250000000001,
1.33303635345042E-32));
#30289=CARTESIAN_POINT('Origin',(-4.38905912375397E-17,-0.0225,1.33303635345025E-32));
#30290=CARTESIAN_POINT('Origin',(-4.38905912375391E-17,-0.02250000000001,
1.33303635345042E-32));
#30291=CARTESIAN_POINT('Origin',(-4.38905912375397E-17,-0.0225,1.33303635345025E-32));
#30292=CARTESIAN_POINT('Origin',(-4.38905912375391E-17,-0.02250000000001,
1.33303635345042E-32));
#30293=CARTESIAN_POINT('Origin',(0.0126071337618777,-0.01,0.00273316269367947));
#30294=CARTESIAN_POINT('Origin',(0.0126071337618875,-0.02250000000001,0.00273316269368159));
#30295=CARTESIAN_POINT('Origin',(-4.38905912375397E-17,-0.0225,1.33303635345025E-32));
#30296=CARTESIAN_POINT('Origin',(-4.38905912375391E-17,-0.02250000000001,
1.33303635345042E-32));
#30297=CARTESIAN_POINT('',(-0.000529682692573584,-0.02250000000001,0.0024432429771081));
#30298=CARTESIAN_POINT('Origin',(-4.38905912375391E-17,-0.02250000000001,
1.33303635345042E-32));
#30299=CARTESIAN_POINT('Origin',(-4.38905912375397E-17,-0.0225,1.33303635345025E-32));
#30300=CARTESIAN_POINT('Origin',(-4.38905912375397E-17,-0.0225,1.33303635345025E-32));
#30301=CARTESIAN_POINT('',(-0.000529682692573584,-0.0225,0.0024432429771081));
#34812=UNCERTAINTY_MEASURE_WITH_UNIT(LENGTH_MEASURE(1.E-5),#34877,
'DISTANCE_ACCURACY_VALUE',
'Maximum model space distance between geometric entities at asserted c
onnectivities');
#34841=UNCERTAINTY_MEASURE_WITH_UNIT(LENGTH_MEASURE(1.E-5),#34877,
'DISTANCE_ACCURACY_VALUE',
'Maximum model space distance between geometric entities at asserted c
onnectivities');
#34847=(
GEOMETRIC_REPRESENTATION_CONTEXT(3)
GLOBAL_UNCERTAINTY_ASSIGNED_CONTEXT((#34812))
GLOBAL_UNIT_ASSIGNED_CONTEXT((#34877,#34878,#34879))
REPRESENTATION_CONTEXT('','3D')
);
#34876=(
GEOMETRIC_REPRESENTATION_CONTEXT(3)
GLOBAL_UNCERTAINTY_ASSIGNED_CONTEXT((#34841))
GLOBAL_UNIT_ASSIGNED_CONTEXT((#34877,#34878,#34879))
REPRESENTATION_CONTEXT('','3D')
);
#34877=(
LENGTH_UNIT()
NAMED_UNIT(*)
SI_UNIT($,.METRE.)
);
#34878=(
NAMED_UNIT(*)
PLANE_ANGLE_UNIT()
SI_UNIT($,.RADIAN.)
);
#34879=(
NAMED_UNIT(*)
SI_UNIT($,.STERADIAN.)
SOLID_ANGLE_UNIT()
);
#34885=SHAPE_DEFINITION_REPRESENTATION(#34919,#34989);
#34919=PRODUCT_DEFINITION_SHAPE('',$,#35024);
#34989=SHAPE_REPRESENTATION('',(#20315),#34847);
#35018=PRODUCT_DEFINITION_CONTEXT('part definition',#35122,'design');
#35024=PRODUCT_DEFINITION('Motor Shaft 1','Motor Shaft 1',#35058,#35018);
#35058=PRODUCT_DEFINITION_FORMATION('',$,#35129);
#35122=APPLICATION_CONTEXT('Managed model based 3d engineering');
#35123=PRODUCT_CONTEXT('part definition',#35122,'mechanical');
#35129=PRODUCT('Motor Shaft 1','Motor Shaft 1',
'LEGAL AND USAGE DISCLAIMER: this Data/Model is provided \X2\201C\X0\A
S IS\X2\201D\X0\ for informational and representational only. It is a 
geometric approximation and is NOT engineered, certified, or guarantee
d for dimensional accuracy, exact tolerances, or production-level prec
ision. Vendor disclaims all implied warranties including fitness for a
 particular purpose. DO NOT USE FOR DIRECT PHYSICAL MANUFACTURING, AUT
OMATED PRODUCTION, OR SAFETY-CRITICAL SYSTEMS without independent engi
neering verification and resolution of any design discrepancies.',(#35123));
#35163=PRESENTATION_STYLE_ASSIGNMENT((#35172));
#35172=SURFACE_STYLE_USAGE(.BOTH.,#35181);
#35181=SURFACE_SIDE_STYLE('',(#35190));
#35190=SURFACE_STYLE_FILL_AREA(#35199);
#35199=FILL_AREA_STYLE('Plastic - Matte (Black)',(#35208));
#35208=FILL_AREA_STYLE_COLOUR('Plastic - Matte (Black)',#35217);
#35217=COLOUR_RGB('Plastic - Matte (Black)',0.0980392156862745,0.0980392156862745,
0.0980392156862745);
ENDSEC;
END-ISO-10303-21;
